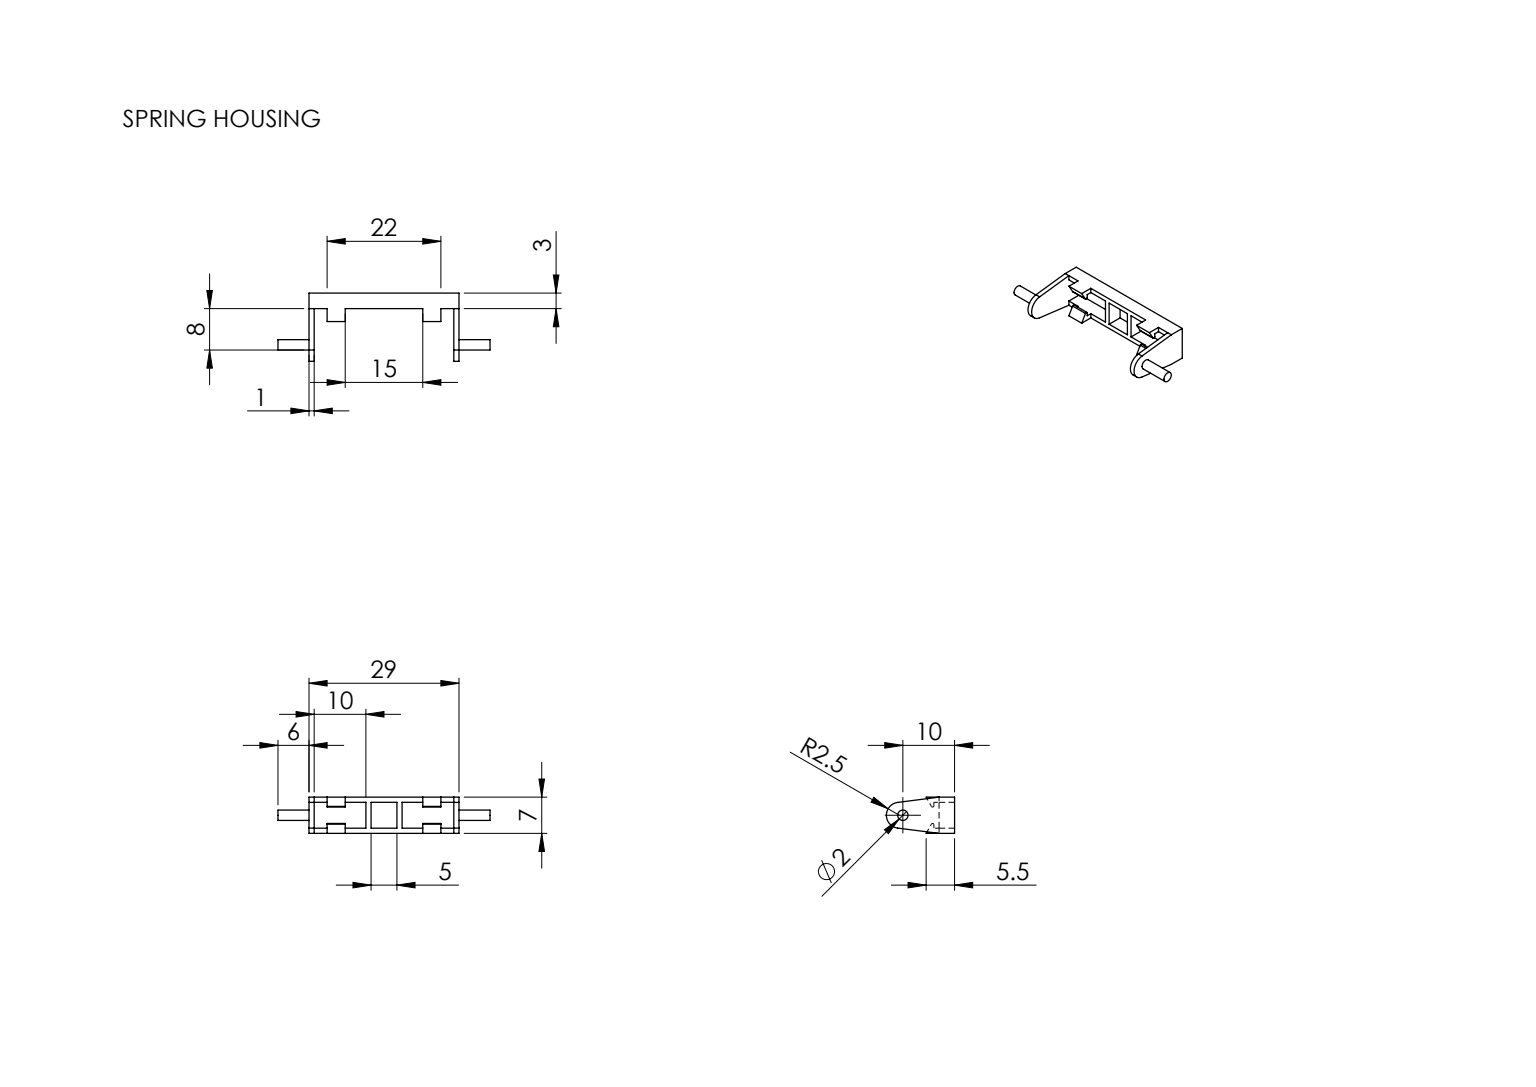
ISO-10303-21;
HEADER;
FILE_DESCRIPTION (('STEP AP214'),
    '1' );
FILE_NAME ('spring housing.step',
    '2026-10-04T16:38:04',
    ( '' ),
    ( '' ),
    'SwSTEP 2.0',
    'SolidWorks 2026',
    '' );
FILE_SCHEMA (( 'AUTOMOTIVE_DESIGN' ));
ENDSEC;

DATA;
#7=VECTOR ( 'NONE', #16168, 1000.000000000000000 ) ;
#16=CARTESIAN_POINT ( 'NONE',  ( -13.49999999999998401, -21.99999999999999645, 11.68378559369222280 ) ) ;
#34=ADVANCED_FACE ( 'NONE', ( #11140 ), #17508, .F. ) ;
#55=EDGE_CURVE ( 'NONE', #14709, #7180, #17615, .T. ) ;
#72=ORIENTED_EDGE ( 'NONE', *, *, #11352, .T. ) ;
#82=EDGE_CURVE ( 'NONE', #4544, #2802, #3495, .T. ) ;
#95=VERTEX_POINT ( 'NONE', #2332 ) ;
#103=LINE ( 'NONE', #17562, #12127 ) ;
#110=CARTESIAN_POINT ( 'NONE',  ( -11.00000000000000000, -25.49999999999999645, 6.500000000000000000 ) ) ;
#154=EDGE_CURVE ( 'NONE', #3175, #3359, #11545, .T. ) ;
#185=FILL_AREA_STYLE ('',( #1857 ) ) ;
#217=ORIENTED_EDGE ( 'NONE', *, *, #4935, .T. ) ;
#220=ORIENTED_EDGE ( 'NONE', *, *, #415, .T. ) ;
#228=DIRECTION ( 'NONE',  ( -0.000000000000000000, -0.000000000000000000, -1.000000000000000000 ) ) ;
#248=EDGE_LOOP ( 'NONE', ( #4182, #12799, #16047, #1135 ) ) ;
#267=ORIENTED_EDGE ( 'NONE', *, *, #11944, .F. ) ;
#268=ORIENTED_EDGE ( 'NONE', *, *, #5212, .F. ) ;
#281=EDGE_CURVE ( 'NONE', #9560, #10619, #19020, .T. ) ;
#292=ORIENTED_EDGE ( 'NONE', *, *, #13482, .F. ) ;
#293=EDGE_CURVE ( 'NONE', #3359, #13135, #6295, .T. ) ;
#296=ORIENTED_EDGE ( 'NONE', *, *, #17959, .F. ) ;
#315=AXIS2_PLACEMENT_3D ( 'NONE', #4243, #16683, #17105 ) ;
#321=CARTESIAN_POINT ( 'NONE',  ( -7.500000000000000000, -20.16506350946107418, 5.000000000000000000 ) ) ;
#332=CARTESIAN_POINT ( 'NONE',  ( -7.500000000000000000, -20.16506350946107418, 5.250000000000000000 ) ) ;
#339=EDGE_CURVE ( 'NONE', #9554, #1664, #7256, .T. ) ;
#354=CARTESIAN_POINT ( 'NONE',  ( -7.499999999999999112, -18.49999999999999645, 4.000000000000000000 ) ) ;
#362=VECTOR ( 'NONE', #20394, 1000.000000000000000 ) ;
#365=CARTESIAN_POINT ( 'NONE',  ( 7.499999999999999112, -23.83493649053891517, 5.249999999999999112 ) ) ;
#372=VECTOR ( 'NONE', #20232, 1000.000000000000000 ) ;
#380=CARTESIAN_POINT ( 'NONE',  ( -7.500000000000000000, -18.49999999999999645, 6.500000000000000888 ) ) ;
#390=DIRECTION ( 'NONE',  ( 0.000000000000000000, 1.000000000000000000, 0.000000000000000000 ) ) ;
#399=ORIENTED_EDGE ( 'NONE', *, *, #570, .F. ) ;
#403=ORIENTED_EDGE ( 'NONE', *, *, #20429, .T. ) ;
#415=EDGE_CURVE ( 'NONE', #11125, #7180, #2437, .T. ) ;
#422=AXIS2_PLACEMENT_3D ( 'NONE', #14755, #433, #5548 ) ;
#433=DIRECTION ( 'NONE',  ( 0.000000000000000000, -0.5000000000000041078, -0.8660254037844363761 ) ) ;
#438=DIRECTION ( 'NONE',  ( -1.000000000000000000, -0.000000000000000000, -0.000000000000000000 ) ) ;
#443=CARTESIAN_POINT ( 'NONE',  ( 11.00000000000000000, -25.49999999999999645, 6.500000000000000000 ) ) ;
#464=AXIS2_PLACEMENT_3D ( 'NONE', #5893, #7568, #2859 ) ;
#467=VECTOR ( 'NONE', #4908, 1000.000000000000000 ) ;
#482=ORIENTED_EDGE ( 'NONE', *, *, #7824, .T. ) ;
#483=VERTEX_POINT ( 'NONE', #11877 ) ;
#528=EDGE_CURVE ( 'NONE', #5816, #15348, #13237, .T. ) ;
#560=DIRECTION ( 'NONE',  ( -0.000000000000000000, 0.000000000000000000, -1.000000000000000000 ) ) ;
#566=EDGE_CURVE ( 'NONE', #17379, #995, #898, .T. ) ;
#570=EDGE_CURVE ( 'NONE', #2226, #5682, #13143, .T. ) ;
#596=CARTESIAN_POINT ( 'NONE',  ( 11.00000000000000000, -18.49999999999999645, 6.500000000000000888 ) ) ;
#608=EDGE_CURVE ( 'NONE', #4592, #5966, #18167, .T. ) ;
#623=DIRECTION ( 'NONE',  ( 0.000000000000000000, 1.000000000000000000, 0.000000000000000000 ) ) ;
#625=VECTOR ( 'NONE', #15350, 1000.000000000000000 ) ;
#635=CARTESIAN_POINT ( 'NONE',  ( -7.500000000000000000, -23.83493649053891517, 4.999999999999999112 ) ) ;
#637=ADVANCED_FACE ( 'NONE', ( #5502 ), #2365, .F. ) ;
#693=DIRECTION ( 'NONE',  ( 1.000000000000000000, 0.000000000000000000, 0.000000000000000000 ) ) ;
#694=CARTESIAN_POINT ( 'NONE',  ( -14.49999999999998579, -18.49999999999999645, 4.000000000000000000 ) ) ;
#716=VECTOR ( 'NONE', #3309, 1000.000000000000000 ) ;
#720=EDGE_CURVE ( 'NONE', #9416, #11125, #2883, .T. ) ;
#735=CARTESIAN_POINT ( 'NONE',  ( 7.499999999999999112, -18.49999999999999645, 6.500000000000000888 ) ) ;
#736=DIRECTION ( 'NONE',  ( 0.000000000000000000, 0.1264857625231113059, 0.9919684228235025047 ) ) ;
#739=CARTESIAN_POINT ( 'NONE',  ( -14.49999999999998579, -25.49999999999999645, 1.000000000000000000 ) ) ;
#741=EDGE_LOOP ( 'NONE', ( #10887, #4261, #18676, #2268, #15145, #1206, #20181, #1106, #10536, #17693, #14548, #16300, #9153, #18986 ) ) ;
#768=ORIENTED_EDGE ( 'NONE', *, *, #15761, .T. ) ;
#790=ORIENTED_EDGE ( 'NONE', *, *, #9633, .T. ) ;
#795=EDGE_CURVE ( 'NONE', #20584, #14806, #3312, .T. ) ;
#809=EDGE_CURVE ( 'NONE', #15986, #11334, #18580, .T. ) ;
#814=VERTEX_POINT ( 'NONE', #10623 ) ;
#838=CARTESIAN_POINT ( 'NONE',  ( -11.00000000000000000, -19.49999999999999645, 5.000000000000000000 ) ) ;
#840=ORIENTED_EDGE ( 'NONE', *, *, #2595, .T. ) ;
#842=VECTOR ( 'NONE', #18531, 1000.000000000000000 ) ;
#858=EDGE_CURVE ( 'NONE', #20067, #12385, #1217, .T. ) ;
#859=DIRECTION ( 'NONE',  ( -1.000000000000000000, 0.000000000000000000, 0.000000000000000000 ) ) ;
#863=ORIENTED_EDGE ( 'NONE', *, *, #1373, .F. ) ;
#867=EDGE_LOOP ( 'NONE', ( #4255, #16725 ) ) ;
#874=CARTESIAN_POINT ( 'NONE',  ( 11.00000000000000000, -24.49999999999999289, 5.000000000000000000 ) ) ;
#891=DIRECTION ( 'NONE',  ( -1.000000000000000000, 0.000000000000000000, 0.000000000000000000 ) ) ;
#896=DIRECTION ( 'NONE',  ( -1.000000000000000000, -0.000000000000000000, -0.000000000000000000 ) ) ;
#898=LINE ( 'NONE', #2062, #2292 ) ;
#914=ORIENTED_EDGE ( 'NONE', *, *, #3010, .F. ) ;
#923=CYLINDRICAL_SURFACE ( 'NONE', #19544, 2.500000000000000444 ) ;
#926=ADVANCED_FACE ( 'NONE', ( #14369 ), #17418, .T. ) ;
#938=LINE ( 'NONE', #739, #9319 ) ;
#948=CARTESIAN_POINT ( 'NONE',  ( 11.00000000000000000, -20.29006350946107418, 5.466506350946110260 ) ) ;
#950=LINE ( 'NONE', #5663, #9851 ) ;
#957=CARTESIAN_POINT ( 'NONE',  ( -11.00000000000000000, -19.49999999999999645, 5.000000000000000000 ) ) ;
#968=VECTOR ( 'NONE', #2534, 1000.000000000000000 ) ;
#973=VECTOR ( 'NONE', #693, 1000.000000000000000 ) ;
#979=CARTESIAN_POINT ( 'NONE',  ( 11.00000000000000000, -18.49999999999999645, 4.000000000000000000 ) ) ;
#987=ADVANCED_FACE ( 'NONE', ( #3397 ), #11143, .F. ) ;
#993=DIRECTION ( 'NONE',  ( -1.000000000000000000, -0.000000000000000000, -0.000000000000000000 ) ) ;
#995=VERTEX_POINT ( 'NONE', #20668 ) ;
#1009=CARTESIAN_POINT ( 'NONE',  ( 7.499999999999999112, -24.49999999999999289, 4.000000000000000000 ) ) ;
#1025=ORIENTED_EDGE ( 'NONE', *, *, #18401, .F. ) ;
#1030=EDGE_CURVE ( 'NONE', #9195, #15413, #4961, .T. ) ;
#1056=( NAMED_UNIT ( * ) PLANE_ANGLE_UNIT ( ) SI_UNIT ( $, .RADIAN. ) );
#1067=LINE ( 'NONE', #9213, #14396 ) ;
#1096=ORIENTED_EDGE ( 'NONE', *, *, #15655, .F. ) ;
#1098=CARTESIAN_POINT ( 'NONE',  ( -13.49999999999998401, -24.49999999999999289, 4.000000000000000000 ) ) ;
#1106=ORIENTED_EDGE ( 'NONE', *, *, #14014, .T. ) ;
#1107=ORIENTED_EDGE ( 'NONE', *, *, #8472, .T. ) ;
#1118=DIRECTION ( 'NONE',  ( -1.000000000000000000, 0.000000000000000000, 0.000000000000000000 ) ) ;
#1120=CARTESIAN_POINT ( 'NONE',  ( -14.49999999999998579, -18.49999999999999645, 4.000000000000000000 ) ) ;
#1122=AXIS2_PLACEMENT_3D ( 'NONE', #3753, #9921, #5424 ) ;
#1135=ORIENTED_EDGE ( 'NONE', *, *, #13755, .F. ) ;
#1158=CARTESIAN_POINT ( 'NONE',  ( -3.499999999999997780, -24.49999999999999289, 4.000000000000000000 ) ) ;
#1159=ORIENTED_EDGE ( 'NONE', *, *, #7829, .F. ) ;
#1160=DIRECTION ( 'NONE',  ( 1.000000000000000000, -0.000000000000000000, -0.000000000000000000 ) ) ;
#1162=CARTESIAN_POINT ( 'NONE',  ( 13.49999999999998401, -21.99999999999999645, 11.68378559369222280 ) ) ;
#1177=ORIENTED_EDGE ( 'NONE', *, *, #15399, .T. ) ;
#1180=VERTEX_POINT ( 'NONE', #19610 ) ;
#1191=CARTESIAN_POINT ( 'NONE',  ( -14.49999999999998579, -25.49999999999999645, 4.000000000000000000 ) ) ;
#1192=LINE ( 'NONE', #9038, #12638 ) ;
#1203=ORIENTED_EDGE ( 'NONE', *, *, #15128, .F. ) ;
#1205=DIRECTION ( 'NONE',  ( -0.000000000000000000, 0.1264857625231113059, -0.9919684228235025047 ) ) ;
#1206=ORIENTED_EDGE ( 'NONE', *, *, #9633, .F. ) ;
#1212=CARTESIAN_POINT ( 'NONE',  ( 13.49999999999998401, -19.52007894294123957, 12.00000000000000000 ) ) ;
#1214=CARTESIAN_POINT ( 'NONE',  ( -14.49999999999998579, -18.49999999999999645, 1.000000000000000000 ) ) ;
#1217=LINE ( 'NONE', #13958, #17678 ) ;
#1232=LINE ( 'NONE', #7714, #19995 ) ;
#1233=ORIENTED_EDGE ( 'NONE', *, *, #720, .F. ) ;
#1243=CARTESIAN_POINT ( 'NONE',  ( 13.49999999999998401, -24.47992105705875332, 12.00000000000000000 ) ) ;
#1263=ORIENTED_EDGE ( 'NONE', *, *, #16479, .T. ) ;
#1292=LINE ( 'NONE', #7570, #4387 ) ;
#1303=VECTOR ( 'NONE', #14815, 1000.000000000000000 ) ;
#1307=CYLINDRICAL_SURFACE ( 'NONE', #12478, 1.000000000000002665 ) ;
#1308=EDGE_CURVE ( 'NONE', #16594, #7416, #10706, .T. ) ;
#1310=VERTEX_POINT ( 'NONE', #2758 ) ;
#1324=VECTOR ( 'NONE', #8795, 1000.000000000000000 ) ;
#1326=CARTESIAN_POINT ( 'NONE',  ( -7.499999999999999112, -18.49999999999999645, 6.500000000000000888 ) ) ;
#1327=DIRECTION ( 'NONE',  ( -1.000000000000000000, 0.000000000000000000, 0.000000000000000000 ) ) ;
#1360=EDGE_CURVE ( 'NONE', #5898, #18235, #5688, .T. ) ;
#1362=EDGE_CURVE ( 'NONE', #8225, #1180, #13727, .T. ) ;
#1373=EDGE_CURVE ( 'NONE', #17295, #15081, #2438, .T. ) ;
#1376=DIRECTION ( 'NONE',  ( -1.000000000000000000, -0.000000000000000000, -0.000000000000000000 ) ) ;
#1390=DIRECTION ( 'NONE',  ( 1.000000000000000000, 0.000000000000000000, -0.000000000000000000 ) ) ;
#1395=CARTESIAN_POINT ( 'NONE',  ( -14.49999999999998579, -21.99999999999999645, 11.68378559369222280 ) ) ;
#1403=EDGE_LOOP ( 'NONE', ( #8385, #4546, #1263, #5932 ) ) ;
#1413=ORIENTED_EDGE ( 'NONE', *, *, #8902, .T. ) ;
#1443=VERTEX_POINT ( 'NONE', #874 ) ;
#1461=VERTEX_POINT ( 'NONE', #20548 ) ;
#1463=ORIENTED_EDGE ( 'NONE', *, *, #2388, .F. ) ;
#1485=ORIENTED_EDGE ( 'NONE', *, *, #20231, .F. ) ;
#1487=ORIENTED_EDGE ( 'NONE', *, *, #4376, .F. ) ;
#1492=EDGE_CURVE ( 'NONE', #8225, #19576, #11119, .T. ) ;
#1495=CARTESIAN_POINT ( 'NONE',  ( -20.49999999999998224, -21.99999999999999645, 11.00000000000000178 ) ) ;
#1505=ORIENTED_EDGE ( 'NONE', *, *, #18166, .T. ) ;
#1508=CARTESIAN_POINT ( 'NONE',  ( 11.00000000000000000, -23.83493649053891517, 4.999999999999999112 ) ) ;
#1514=DIRECTION ( 'NONE',  ( 1.000000000000000000, 0.000000000000000000, 0.000000000000000000 ) ) ;
#1534=ORIENTED_EDGE ( 'NONE', *, *, #3010, .T. ) ;
#1538=EDGE_CURVE ( 'NONE', #2967, #1461, #17489, .T. ) ;
#1553=ORIENTED_EDGE ( 'NONE', *, *, #6829, .T. ) ;
#1554=AXIS2_PLACEMENT_3D ( 'NONE', #19099, #8305, #11236 ) ;
#1570=EDGE_CURVE ( 'NONE', #1664, #16077, #9543, .T. ) ;
#1575=CARTESIAN_POINT ( 'NONE',  ( -14.49999999999998579, -25.49999999999999645, 4.000000000000000000 ) ) ;
#1582=PLANE ( 'NONE',  #7681 ) ;
#1596=EDGE_CURVE ( 'NONE', #2802, #18601, #3387, .T. ) ;
#1616=DIRECTION ( 'NONE',  ( 0.000000000000000000, 0.000000000000000000, 1.000000000000000000 ) ) ;
#1627=VECTOR ( 'NONE', #3594, 1000.000000000000000 ) ;
#1639=CARTESIAN_POINT ( 'NONE',  ( 7.499999999999999112, -20.16506350946107418, 5.000000000000000000 ) ) ;
#1650=DIRECTION ( 'NONE',  ( 0.000000000000000000, 0.1264857625231113059, 0.9919684228235025047 ) ) ;
#1654=CARTESIAN_POINT ( 'NONE',  ( 11.00000000000000000, -18.49999999999999645, 6.500000000000000888 ) ) ;
#1663=VECTOR ( 'NONE', #13515, 1000.000000000000000 ) ;
#1664=VERTEX_POINT ( 'NONE', #443 ) ;
#1669=CARTESIAN_POINT ( 'NONE',  ( 11.00000000000000000, -20.16506350946107418, 5.000000000000000000 ) ) ;
#1698=DIRECTION ( 'NONE',  ( -1.000000000000000000, 0.000000000000000000, 0.000000000000000000 ) ) ;
#1709=EDGE_CURVE ( 'NONE', #17379, #20661, #13091, .T. ) ;
#1713=CARTESIAN_POINT ( 'NONE',  ( 13.49999999999998401, -19.52007894294123957, 12.00000000000000000 ) ) ;
#1724=CARTESIAN_POINT ( 'NONE',  ( 7.499999999999999112, -23.83493649053891517, 4.999999999999999112 ) ) ;
#1732=EDGE_CURVE ( 'NONE', #3797, #7379, #13191, .T. ) ;
#1771=CIRCLE ( 'NONE', #7777, 1.000000000000002665 ) ;
#1785=DIRECTION ( 'NONE',  ( 0.000000000000000000, 0.000000000000000000, 1.000000000000000000 ) ) ;
#1790=ORIENTED_EDGE ( 'NONE', *, *, #11684, .T. ) ;
#1793=CARTESIAN_POINT ( 'NONE',  ( 0.000000000000000000, 0.000000000000000000, 0.000000000000000000 ) ) ;
#1797=CARTESIAN_POINT ( 'NONE',  ( 14.50000000000001243, -18.49999999999999645, 1.000000000000000000 ) ) ;
#1803=DIRECTION ( 'NONE',  ( -1.000000000000000000, -0.000000000000000000, -0.000000000000000000 ) ) ;
#1806=EDGE_CURVE ( 'NONE', #3359, #14333, #8700, .T. ) ;
#1823=DIRECTION ( 'NONE',  ( -0.000000000000000000, 0.000000000000000000, 1.000000000000000000 ) ) ;
#1824=ORIENTED_EDGE ( 'NONE', *, *, #16454, .T. ) ;
#1826=CARTESIAN_POINT ( 'NONE',  ( 11.00000000000000000, -20.16506350946107418, 5.000000000000000000 ) ) ;
#1836=ORIENTED_EDGE ( 'NONE', *, *, #5658, .T. ) ;
#1857=FILL_AREA_STYLE_COLOUR ( '', #17300 ) ;
#1859=PLANE ( 'NONE',  #6196 ) ;
#1871=ORIENTED_EDGE ( 'NONE', *, *, #10640, .F. ) ;
#1888=PLANE ( 'NONE',  #11720 ) ;
#1899=CARTESIAN_POINT ( 'NONE',  ( -13.49999999999998401, -21.99999999999999645, 14.18378559369222280 ) ) ;
#1910=AXIS2_PLACEMENT_3D ( 'NONE', #9537, #3065, #12980 ) ;
#1912=DIRECTION ( 'NONE',  ( 1.734723475976809560E-16, -1.000000000000000000, 0.000000000000000000 ) ) ;
#1923=PLANE ( 'NONE',  #2904 ) ;
#1929=AXIS2_PLACEMENT_3D ( 'NONE', #10642, #15450, #16810 ) ;
#1941=DIRECTION ( 'NONE',  ( -0.000000000000000000, -0.8660254037844364872, -0.5000000000000036637 ) ) ;
#1950=VECTOR ( 'NONE', #12612, 1000.000000000000000 ) ;
#1958=SURFACE_SIDE_STYLE ('',( #8035 ) ) ;
#1960=DIRECTION ( 'NONE',  ( -0.000000000000000000, 0.000000000000000000, -1.000000000000000000 ) ) ;
#1974=AXIS2_PLACEMENT_3D ( 'NONE', #12021, #11711, #18107 ) ;
#1977=EDGE_CURVE ( 'NONE', #7180, #17356, #1067, .T. ) ;
#1996=ORIENTED_EDGE ( 'NONE', *, *, #15355, .T. ) ;
#1998=DIRECTION ( 'NONE',  ( -0.000000000000000000, -0.000000000000000000, -1.000000000000000000 ) ) ;
#2013=FACE_BOUND ( 'NONE', #12922, .T. ) ;
#2029=LINE ( 'NONE', #8418, #8249 ) ;
#2037=VECTOR ( 'NONE', #17601, 1000.000000000000000 ) ;
#2049=ORIENTED_EDGE ( 'NONE', *, *, #17282, .T. ) ;
#2054=DIRECTION ( 'NONE',  ( -1.000000000000000000, -0.000000000000000000, -0.000000000000000000 ) ) ;
#2062=CARTESIAN_POINT ( 'NONE',  ( 7.500000000000000000, -19.49999999999999645, 4.000000000000000000 ) ) ;
#2082=ORIENTED_EDGE ( 'NONE', *, *, #12798, .F. ) ;
#2087=CARTESIAN_POINT ( 'NONE',  ( 0.000000000000000000, 0.000000000000000000, 1.000000000000000000 ) ) ;
#2089=DIRECTION ( 'NONE',  ( -1.000000000000000000, -0.000000000000000000, -0.000000000000000000 ) ) ;
#2102=CARTESIAN_POINT ( 'NONE',  ( -11.00000000000000000, -23.83493649053891517, 4.999999999999999112 ) ) ;
#2109=EDGE_CURVE ( 'NONE', #13777, #3840, #4508, .T. ) ;
#2116=CARTESIAN_POINT ( 'NONE',  ( -14.49999999999998579, -21.99999999999999645, 11.68378559369222280 ) ) ;
#2127=VERTEX_POINT ( 'NONE', #9728 ) ;
#2130=PLANE ( 'NONE',  #19291 ) ;
#2136=CARTESIAN_POINT ( 'NONE',  ( 7.499999999999999112, -19.49999999999999645, 4.000000000000000000 ) ) ;
#2157=CYLINDRICAL_SURFACE ( 'NONE', #20022, 2.500000000000000444 ) ;
#2171=EDGE_CURVE ( 'NONE', #5966, #15986, #11290, .T. ) ;
#2176=DIRECTION ( 'NONE',  ( -0.000000000000000000, -1.000000000000000000, 0.000000000000000000 ) ) ;
#2178=CIRCLE ( 'NONE', #12865, 1.000000000000002665 ) ;
#2186=CARTESIAN_POINT ( 'NONE',  ( -14.49999999999998579, -21.99999999999999645, 11.00000000000000178 ) ) ;
#2190=LINE ( 'NONE', #10147, #4721 ) ;
#2203=EDGE_CURVE ( 'NONE', #17464, #10229, #7754, .T. ) ;
#2208=CARTESIAN_POINT ( 'NONE',  ( 11.00000000000000000, -20.16506350946107418, 5.250000000000000000 ) ) ;
#2226=VERTEX_POINT ( 'NONE', #110 ) ;
#2232=DIRECTION ( 'NONE',  ( 0.000000000000000000, -0.1264857625231113059, 0.9919684228235025047 ) ) ;
#2250=ORIENTED_EDGE ( 'NONE', *, *, #19877, .T. ) ;
#2255=CARTESIAN_POINT ( 'NONE',  ( -11.00000000000000000, -20.16506350946107418, 5.000000000000000000 ) ) ;
#2268=ORIENTED_EDGE ( 'NONE', *, *, #2171, .F. ) ;
#2270=PLANE ( 'NONE',  #1929 ) ;
#2275=ORIENTED_EDGE ( 'NONE', *, *, #1977, .F. ) ;
#2292=VECTOR ( 'NONE', #11978, 1000.000000000000000 ) ;
#2296=VERTEX_POINT ( 'NONE', #5326 ) ;
#2297=VERTEX_POINT ( 'NONE', #3653 ) ;
#2301=CARTESIAN_POINT ( 'NONE',  ( -14.49999999999998579, -24.49999999999999289, 4.000000000000000000 ) ) ;
#2330=VECTOR ( 'NONE', #7851, 1000.000000000000000 ) ;
#2332=CARTESIAN_POINT ( 'NONE',  ( -7.499999999999999112, -24.49999999999999289, 4.000000000000000000 ) ) ;
#2352=EDGE_CURVE ( 'NONE', #14282, #12772, #12019, .T. ) ;
#2362=EDGE_CURVE ( 'NONE', #12874, #9416, #3451, .T. ) ;
#2365=PLANE ( 'NONE',  #17326 ) ;
#2367=DIRECTION ( 'NONE',  ( 1.000000000000000000, 0.000000000000000000, 0.000000000000000000 ) ) ;
#2385=ORIENTED_EDGE ( 'NONE', *, *, #2109, .F. ) ;
#2388=EDGE_CURVE ( 'NONE', #814, #18396, #10689, .T. ) ;
#2393=CARTESIAN_POINT ( 'NONE',  ( -13.49999999999998401, -19.52007894294123957, 12.00000000000000000 ) ) ;
#2394=CARTESIAN_POINT ( 'NONE',  ( 13.50000000000001243, -18.49999999999999645, 4.000000000000000000 ) ) ;
#2400=DIRECTION ( 'NONE',  ( 0.000000000000000000, -0.8660254037844363761, 0.5000000000000041078 ) ) ;
#2430=CARTESIAN_POINT ( 'NONE',  ( 20.49999999999998224, -21.99999999999999645, 9.999999999999998224 ) ) ;
#2434=DIRECTION ( 'NONE',  ( 1.000000000000000000, 0.000000000000000000, -0.000000000000000000 ) ) ;
#2437=LINE ( 'NONE', #15195, #968 ) ;
#2438=LINE ( 'NONE', #18867, #372 ) ;
#2456=ADVANCED_FACE ( 'NONE', ( #19567 ), #8167, .T. ) ;
#2457=ORIENTED_EDGE ( 'NONE', *, *, #4151, .T. ) ;
#2484=DIRECTION ( 'NONE',  ( 0.000000000000000000, 1.000000000000000000, 0.000000000000000000 ) ) ;
#2494=PLANE ( 'NONE',  #20651 ) ;
#2495=CARTESIAN_POINT ( 'NONE',  ( 11.00000000000000000, -24.49999999999999289, 5.000000000000000000 ) ) ;
#2510=CARTESIAN_POINT ( 'NONE',  ( -14.49999999999998579, -24.49999999999999289, 1.000000000000000000 ) ) ;
#2512=VECTOR ( 'NONE', #15224, 1000.000000000000000 ) ;
#2515=ADVANCED_FACE ( 'NONE', ( #16604 ), #7212, .T. ) ;
#2534=DIRECTION ( 'NONE',  ( -0.000000000000000000, -0.000000000000000000, -1.000000000000000000 ) ) ;
#2561=ORIENTED_EDGE ( 'NONE', *, *, #16454, .F. ) ;
#2569=CARTESIAN_POINT ( 'NONE',  ( -14.49999999999998579, -19.49999999999999645, 4.000000000000000000 ) ) ;
#2585=ORIENTED_EDGE ( 'NONE', *, *, #14183, .T. ) ;
#2587=ORIENTED_EDGE ( 'NONE', *, *, #10224, .T. ) ;
#2595=EDGE_CURVE ( 'NONE', #7178, #9560, #20082, .T. ) ;
#2602=DIRECTION ( 'NONE',  ( 0.000000000000000000, 0.8660254037844363761, -0.5000000000000041078 ) ) ;
#2612=VECTOR ( 'NONE', #15562, 1000.000000000000000 ) ;
#2613=DIRECTION ( 'NONE',  ( 0.000000000000000000, 0.000000000000000000, -1.000000000000000000 ) ) ;
#2623=AXIS2_PLACEMENT_3D ( 'NONE', #3905, #10283, #16654 ) ;
#2627=CIRCLE ( 'NONE', #16989, 0.2500000000000002220 ) ;
#2641=VECTOR ( 'NONE', #4244, 1000.000000000000114 ) ;
#2648=CARTESIAN_POINT ( 'NONE',  ( 2.499999999999998668, -19.49999999999999645, 4.000000000000000000 ) ) ;
#2673=DIRECTION ( 'NONE',  ( 0.000000000000000000, 0.000000000000000000, -1.000000000000000000 ) ) ;
#2680=VECTOR ( 'NONE', #5272, 1000.000000000000000 ) ;
#2694=CARTESIAN_POINT ( 'NONE',  ( 2.499999999999998668, -19.50000000000000000, 1.000000000000000000 ) ) ;
#2703=EDGE_CURVE ( 'NONE', #14026, #15081, #10766, .T. ) ;
#2715=DIRECTION ( 'NONE',  ( 1.000000000000000000, 0.000000000000000000, -0.000000000000000000 ) ) ;
#2742=VECTOR ( 'NONE', #6065, 1000.000000000000227 ) ;
#2758=CARTESIAN_POINT ( 'NONE',  ( 13.50000000000001243, -24.49999999999999289, 1.000000000000000000 ) ) ;
#2765=ORIENTED_EDGE ( 'NONE', *, *, #9898, .T. ) ;
#2778=ORIENTED_EDGE ( 'NONE', *, *, #293, .F. ) ;
#2785=FACE_BOUND ( 'NONE', #9102, .T. ) ;
#2802=VERTEX_POINT ( 'NONE', #13122 ) ;
#2815=DIRECTION ( 'NONE',  ( 0.000000000000000000, 0.8660254037844364872, 0.5000000000000036637 ) ) ;
#2825=EDGE_LOOP ( 'NONE', ( #1203, #14184, #13332, #8079, #16097, #14135 ) ) ;
#2826=ORIENTED_EDGE ( 'NONE', *, *, #17610, .T. ) ;
#2859=DIRECTION ( 'NONE',  ( 0.000000000000000000, 0.000000000000000000, -1.000000000000000000 ) ) ;
#2861=EDGE_CURVE ( 'NONE', #14282, #483, #9781, .T. ) ;
#2865=EDGE_LOOP ( 'NONE', ( #2826, #2049, #1487, #13747 ) ) ;
#2870=ORIENTED_EDGE ( 'NONE', *, *, #2861, .F. ) ;
#2883=LINE ( 'NONE', #12188, #6992 ) ;
#2896=EDGE_CURVE ( 'NONE', #20148, #17464, #8426, .T. ) ;
#2904=AXIS2_PLACEMENT_3D ( 'NONE', #3090, #1823, #1514 ) ;
#2919=LINE ( 'NONE', #4586, #17101 ) ;
#2946=FACE_OUTER_BOUND ( 'NONE', #3035, .T. ) ;
#2949=ORIENTED_EDGE ( 'NONE', *, *, #3053, .F. ) ;
#2960=CYLINDRICAL_SURFACE ( 'NONE', #3344, 1.000000000000002665 ) ;
#2967=VERTEX_POINT ( 'NONE', #1797 ) ;
#2985=ORIENTED_EDGE ( 'NONE', *, *, #1362, .F. ) ;
#2988=AXIS2_PLACEMENT_3D ( 'NONE', #3732, #13144, #11263 ) ;
#2992=CARTESIAN_POINT ( 'NONE',  ( 11.00000000000000000, -19.49999999999999645, 4.000000000000000000 ) ) ;
#2995=DIRECTION ( 'NONE',  ( -1.000000000000000000, -0.000000000000000000, -0.000000000000000000 ) ) ;
#3010=EDGE_CURVE ( 'NONE', #11512, #8225, #8280, .T. ) ;
#3016=AXIS2_PLACEMENT_3D ( 'NONE', #2394, #10656, #18716 ) ;
#3021=VECTOR ( 'NONE', #1650, 1000.000000000000227 ) ;
#3027=DIRECTION ( 'NONE',  ( -0.000000000000000000, 0.000000000000000000, -1.000000000000000000 ) ) ;
#3034=CARTESIAN_POINT ( 'NONE',  ( 11.00000000000000000, -23.83493649053891517, 5.249999999999999112 ) ) ;
#3035=EDGE_LOOP ( 'NONE', ( #2082, #7589, #3333, #14527 ) ) ;
#3038=EDGE_CURVE ( 'NONE', #2127, #18601, #16130, .T. ) ;
#3053=EDGE_CURVE ( 'NONE', #5903, #4592, #11310, .T. ) ;
#3055=LINE ( 'NONE', #15801, #10085 ) ;
#3061=VERTEX_POINT ( 'NONE', #14652 ) ;
#3065=DIRECTION ( 'NONE',  ( -1.000000000000000000, -0.000000000000000000, -0.000000000000000000 ) ) ;
#3068=DIRECTION ( 'NONE',  ( -0.000000000000000000, -0.000000000000000000, -1.000000000000000000 ) ) ;
#3078=DIRECTION ( 'NONE',  ( 0.000000000000000000, -0.1264857625231113059, -0.9919684228235025047 ) ) ;
#3090=CARTESIAN_POINT ( 'NONE',  ( 0.000000000000000000, 0.000000000000000000, 4.000000000000000000 ) ) ;
#3105=EDGE_CURVE ( 'NONE', #13135, #11513, #19380, .T. ) ;
#3109=LINE ( 'NONE', #7816, #19369 ) ;
#3121=CARTESIAN_POINT ( 'NONE',  ( -13.49999999999998401, -25.49999999999999645, 4.000000000000000000 ) ) ;
#3123=CARTESIAN_POINT ( 'NONE',  ( -14.49999999999998579, -19.49999999999999645, 4.000000000000000000 ) ) ;
#3139=AXIS2_PLACEMENT_3D ( 'NONE', #10187, #16557, #2232 ) ;
#3162=ORIENTED_EDGE ( 'NONE', *, *, #9798, .F. ) ;
#3163=CARTESIAN_POINT ( 'NONE',  ( -7.500000000000000000, -20.29006350946107418, 5.466506350946110260 ) ) ;
#3175=VERTEX_POINT ( 'NONE', #14760 ) ;
#3180=ORIENTED_EDGE ( 'NONE', *, *, #17282, .F. ) ;
#3187=AXIS2_PLACEMENT_3D ( 'NONE', #9363, #16628, #4194 ) ;
#3195=DIRECTION ( 'NONE',  ( 1.000000000000000000, 8.673617379884045333E-17, -0.000000000000000000 ) ) ;
#3206=ORIENTED_EDGE ( 'NONE', *, *, #7111, .F. ) ;
#3231=DIRECTION ( 'NONE',  ( 0.000000000000000000, -1.000000000000000000, 0.000000000000000000 ) ) ;
#3261=CYLINDRICAL_SURFACE ( 'NONE', #1910, 1.000000000000002665 ) ;
#3272=ORIENTED_EDGE ( 'NONE', *, *, #339, .F. ) ;
#3285=AXIS2_PLACEMENT_3D ( 'NONE', #18381, #18068, #2367 ) ;
#3286=CARTESIAN_POINT ( 'NONE',  ( 11.00000000000000000, -23.83493649053891517, 5.249999999999999112 ) ) ;
#3295=AXIS2_PLACEMENT_3D ( 'NONE', #17829, #13417, #14883 ) ;
#3296=CIRCLE ( 'NONE', #5975, 1.000000000000002665 ) ;
#3309=DIRECTION ( 'NONE',  ( -0.000000000000000000, -1.000000000000000000, 0.000000000000000000 ) ) ;
#3312=CIRCLE ( 'NONE', #4652, 1.000000000000002665 ) ;
#3315=DIRECTION ( 'NONE',  ( -1.000000000000000000, 0.000000000000000000, 0.000000000000000000 ) ) ;
#3324=ORIENTED_EDGE ( 'NONE', *, *, #20088, .T. ) ;
#3332=CIRCLE ( 'NONE', #11346, 2.500000000000000444 ) ;
#3333=ORIENTED_EDGE ( 'NONE', *, *, #2896, .T. ) ;
#3336=ORIENTED_EDGE ( 'NONE', *, *, #17550, .T. ) ;
#3344=AXIS2_PLACEMENT_3D ( 'NONE', #1495, #20449, #14143 ) ;
#3359=VERTEX_POINT ( 'NONE', #635 ) ;
#3387=CIRCLE ( 'NONE', #19421, 2.500000000000000444 ) ;
#3395=VERTEX_POINT ( 'NONE', #15064 ) ;
#3397=FACE_OUTER_BOUND ( 'NONE', #13302, .T. ) ;
#3414=ORIENTED_EDGE ( 'NONE', *, *, #10183, .T. ) ;
#3416=CARTESIAN_POINT ( 'NONE',  ( -3.499999999999997780, -19.49999999999999645, 4.000000000000000000 ) ) ;
#3420=ORIENTED_EDGE ( 'NONE', *, *, #720, .T. ) ;
#3437=VERTEX_POINT ( 'NONE', #1326 ) ;
#3439=CARTESIAN_POINT ( 'NONE',  ( 2.499999999999999112, -24.49999999999999289, 1.000000000000000000 ) ) ;
#3448=PLANE ( 'NONE',  #14464 ) ;
#3451=LINE ( 'NONE', #3861, #20059 ) ;
#3456=LINE ( 'NONE', #14636, #18079 ) ;
#3461=ORIENTED_EDGE ( 'NONE', *, *, #13218, .T. ) ;
#3482=EDGE_CURVE ( 'NONE', #1664, #11612, #15539, .T. ) ;
#3494=CARTESIAN_POINT ( 'NONE',  ( 14.50000000000001243, -25.49999999999999645, 4.000000000000000000 ) ) ;
#3495=LINE ( 'NONE', #9974, #10646 ) ;
#3501=CARTESIAN_POINT ( 'NONE',  ( -14.49999999999998579, -19.49999999999999645, 1.000000000000000000 ) ) ;
#3511=AXIS2_PLACEMENT_3D ( 'NONE', #2208, #15069, #8590 ) ;
#3530=LINE ( 'NONE', #3123, #3940 ) ;
#3532=CARTESIAN_POINT ( 'NONE',  ( 11.00000000000000000, -20.16506350946107418, 5.250000000000000000 ) ) ;
#3538=ORIENTED_EDGE ( 'NONE', *, *, #2203, .T. ) ;
#3541=ORIENTED_EDGE ( 'NONE', *, *, #10425, .T. ) ;
#3544=PLANE ( 'NONE',  #1122 ) ;
#3556=PLANE ( 'NONE',  #8080 ) ;
#3594=DIRECTION ( 'NONE',  ( 0.000000000000000000, 1.000000000000000000, -1.304178812473495102E-15 ) ) ;
#3610=CARTESIAN_POINT ( 'NONE',  ( -11.00000000000000000, -23.70993649053891517, 5.466506350946108483 ) ) ;
#3613=CARTESIAN_POINT ( 'NONE',  ( 7.499999999999999112, -18.49999999999999645, 4.000000000000000000 ) ) ;
#3643=SHAPE_DEFINITION_REPRESENTATION ( #5005, #6161 ) ;
#3653=CARTESIAN_POINT ( 'NONE',  ( -2.499999999999998668, -24.49999999999999289, 4.000000000000000000 ) ) ;
#3668=DIRECTION ( 'NONE',  ( 1.734723475976809560E-16, -1.000000000000000000, 0.000000000000000000 ) ) ;
#3672=VECTOR ( 'NONE', #7591, 1000.000000000000000 ) ;
#3697=ORIENTED_EDGE ( 'NONE', *, *, #7459, .F. ) ;
#3698=EDGE_LOOP ( 'NONE', ( #10786, #8846, #17765, #2870 ) ) ;
#3732=CARTESIAN_POINT ( 'NONE',  ( 11.00000000000000000, -23.83493649053891517, 4.999999999999999112 ) ) ;
#3751=VERTEX_POINT ( 'NONE', #6113 ) ;
#3753=CARTESIAN_POINT ( 'NONE',  ( -11.00000000000000000, -23.83493649053891517, 5.249999999999999112 ) ) ;
#3759=CARTESIAN_POINT ( 'NONE',  ( -14.49999999999998579, -19.49999999999999645, 1.000000000000000000 ) ) ;
#3769=AXIS2_PLACEMENT_3D ( 'NONE', #9130, #2434, #5887 ) ;
#3775=DIRECTION ( 'NONE',  ( 0.000000000000000000, 0.000000000000000000, -1.000000000000000000 ) ) ;
#3797=VERTEX_POINT ( 'NONE', #1098 ) ;
#3800=DIRECTION ( 'NONE',  ( -0.000000000000000000, -0.8660254037844363761, 0.5000000000000041078 ) ) ;
#3809=PLANE ( 'NONE',  #3139 ) ;
#3815=ORIENTED_EDGE ( 'NONE', *, *, #12646, .T. ) ;
#3825=FACE_OUTER_BOUND ( 'NONE', #867, .T. ) ;
#3831=FACE_OUTER_BOUND ( 'NONE', #4590, .T. ) ;
#3840=VERTEX_POINT ( 'NONE', #20142 ) ;
#3857=DIRECTION ( 'NONE',  ( -0.000000000000000000, -0.000000000000000000, 1.000000000000000000 ) ) ;
#3861=CARTESIAN_POINT ( 'NONE',  ( -14.49999999999998579, -18.49999999999999645, 4.000000000000000000 ) ) ;
#3873=PLANE ( 'NONE',  #422 ) ;
#3886=FACE_OUTER_BOUND ( 'NONE', #6170, .T. ) ;
#3900=ADVANCED_FACE ( 'NONE', ( #5900 ), #12270, .T. ) ;
#3905=CARTESIAN_POINT ( 'NONE',  ( -7.500000000000000000, -23.83493649053891517, 5.249999999999999112 ) ) ;
#3914=ORIENTED_EDGE ( 'NONE', *, *, #2703, .T. ) ;
#3932=FACE_OUTER_BOUND ( 'NONE', #14417, .T. ) ;
#3933=ADVANCED_FACE ( 'NONE', ( #9145 ), #6005, .T. ) ;
#3940=VECTOR ( 'NONE', #9905, 1000.000000000000000 ) ;
#3947=CARTESIAN_POINT ( 'NONE',  ( 11.00000000000000000, -20.16506350946107418, 5.000000000000000000 ) ) ;
#3953=DIRECTION ( 'NONE',  ( 0.000000000000000000, 0.000000000000000000, 1.000000000000000000 ) ) ;
#3964=DIRECTION ( 'NONE',  ( -0.000000000000000000, 0.000000000000000000, -1.000000000000000000 ) ) ;
#3965=DIRECTION ( 'NONE',  ( 0.000000000000000000, -0.5000000000000041078, -0.8660254037844363761 ) ) ;
#3970=LINE ( 'NONE', #838, #1324 ) ;
#3976=VECTOR ( 'NONE', #2484, 1000.000000000000000 ) ;
#3978=FILL_AREA_STYLE_COLOUR ( '', #19719 ) ;
#3994=CARTESIAN_POINT ( 'NONE',  ( -14.49999999999998579, -19.49999999999999645, 4.000000000000000000 ) ) ;
#4007=DIRECTION ( 'NONE',  ( -1.000000000000000000, 0.000000000000000000, 0.000000000000000000 ) ) ;
#4023=VECTOR ( 'NONE', #12979, 1000.000000000000000 ) ;
#4063=ORIENTED_EDGE ( 'NONE', *, *, #4119, .T. ) ;
#4074=ORIENTED_EDGE ( 'NONE', *, *, #18619, .F. ) ;
#4094=VECTOR ( 'NONE', #17098, 1000.000000000000000 ) ;
#4119=EDGE_CURVE ( 'NONE', #8041, #16594, #9859, .T. ) ;
#4142=DIRECTION ( 'NONE',  ( 0.000000000000000000, 0.000000000000000000, 1.000000000000000000 ) ) ;
#4151=EDGE_CURVE ( 'NONE', #14709, #13797, #4844, .T. ) ;
#4159=CARTESIAN_POINT ( 'NONE',  ( 3.499999999999998668, -24.49999999999999289, 1.000000000000000000 ) ) ;
#4182=ORIENTED_EDGE ( 'NONE', *, *, #5534, .F. ) ;
#4194=DIRECTION ( 'NONE',  ( 0.000000000000000000, 0.000000000000000000, -1.000000000000000000 ) ) ;
#4218=LINE ( 'NONE', #7470, #8160 ) ;
#4220=DIRECTION ( 'NONE',  ( 0.000000000000000000, 0.000000000000000000, 1.000000000000000000 ) ) ;
#4235=ORIENTED_EDGE ( 'NONE', *, *, #4541, .F. ) ;
#4243=CARTESIAN_POINT ( 'NONE',  ( -14.49999999999998579, -18.49999999999999645, 4.000000000000000000 ) ) ;
#4244=DIRECTION ( 'NONE',  ( -0.000000000000000000, -0.8660254037844364872, -0.5000000000000036637 ) ) ;
#4255=ORIENTED_EDGE ( 'NONE', *, *, #9260, .T. ) ;
#4261=ORIENTED_EDGE ( 'NONE', *, *, #12949, .T. ) ;
#4282=ORIENTED_EDGE ( 'NONE', *, *, #13693, .T. ) ;
#4288=CIRCLE ( 'NONE', #12301, 1.000000000000002665 ) ;
#4305=DIRECTION ( 'NONE',  ( 0.000000000000000000, -0.8660254037844364872, -0.5000000000000036637 ) ) ;
#4342=LINE ( 'NONE', #8179, #4094 ) ;
#4376=EDGE_CURVE ( 'NONE', #9554, #3751, #13120, .T. ) ;
#4387=VECTOR ( 'NONE', #11954, 1000.000000000000000 ) ;
#4391=CARTESIAN_POINT ( 'NONE',  ( -7.500000000000000000, -25.49999999999999645, 6.500000000000000000 ) ) ;
#4395=EDGE_LOOP ( 'NONE', ( #863, #72, #15191, #3914 ) ) ;
#4406=DIRECTION ( 'NONE',  ( 0.000000000000000000, 0.000000000000000000, 1.000000000000000000 ) ) ;
#4421=ORIENTED_EDGE ( 'NONE', *, *, #14210, .F. ) ;
#4448=ORIENTED_EDGE ( 'NONE', *, *, #2388, .T. ) ;
#4451=CARTESIAN_POINT ( 'NONE',  ( -13.49999999999998401, -18.49999999999999645, 4.000000000000000000 ) ) ;
#4457=CARTESIAN_POINT ( 'NONE',  ( -3.499999999999998668, -19.50000000000000000, 1.000000000000000000 ) ) ;
#4462=AXIS2_PLACEMENT_3D ( 'NONE', #9255, #8666, #15626 ) ;
#4477=ORIENTED_EDGE ( 'NONE', *, *, #9972, .T. ) ;
#4488=ORIENTED_EDGE ( 'NONE', *, *, #15399, .F. ) ;
#4499=SHAPE_REPRESENTATION_RELATIONSHIP ( 'NONE' , 'NONE' ,  #6161, #10808 ) ;
#4508=LINE ( 'NONE', #14016, #6343 ) ;
#4541=EDGE_CURVE ( 'NONE', #13777, #1443, #1292, .T. ) ;
#4544=VERTEX_POINT ( 'NONE', #1191 ) ;
#4546=ORIENTED_EDGE ( 'NONE', *, *, #19785, .F. ) ;
#4550=LINE ( 'NONE', #9358, #12797 ) ;
#4586=CARTESIAN_POINT ( 'NONE',  ( 7.500000000000000000, -24.49999999999999289, 4.000000000000000000 ) ) ;
#4589=CARTESIAN_POINT ( 'NONE',  ( 14.50000000000001243, -25.49999999999999645, 1.000000000000000000 ) ) ;
#4590=EDGE_LOOP ( 'NONE', ( #7386, #18778, #10107, #12587 ) ) ;
#4592=VERTEX_POINT ( 'NONE', #979 ) ;
#4599=AXIS2_PLACEMENT_3D ( 'NONE', #6598, #19668, #19782 ) ;
#4609=MECHANICAL_DESIGN_GEOMETRIC_PRESENTATION_REPRESENTATION('',(#8290),#10966);
#4615=ORIENTED_EDGE ( 'NONE', *, *, #13480, .T. ) ;
#4616=CARTESIAN_POINT ( 'NONE',  ( 7.499999999999999112, -18.49999999999999645, 6.500000000000000888 ) ) ;
#4617=FACE_OUTER_BOUND ( 'NONE', #13878, .T. ) ;
#4622=VECTOR ( 'NONE', #8903, 1000.000000000000000 ) ;
#4638=VECTOR ( 'NONE', #10343, 1000.000000000000000 ) ;
#4643=ORIENTED_EDGE ( 'NONE', *, *, #13693, .F. ) ;
#4652=AXIS2_PLACEMENT_3D ( 'NONE', #6130, #1118, #13757 ) ;
#4654=FACE_OUTER_BOUND ( 'NONE', #1403, .T. ) ;
#4655=DIRECTION ( 'NONE',  ( 0.000000000000000000, 0.000000000000000000, -1.000000000000000000 ) ) ;
#4657=CARTESIAN_POINT ( 'NONE',  ( -7.499999999999999112, -19.49999999999999645, 4.000000000000000000 ) ) ;
#4683=CARTESIAN_POINT ( 'NONE',  ( -20.49999999999998224, -21.99999999999999645, 9.999999999999998224 ) ) ;
#4705=CARTESIAN_POINT ( 'NONE',  ( 11.00000000000000000, -25.49999999999999645, 4.000000000000000000 ) ) ;
#4721=VECTOR ( 'NONE', #1785, 1000.000000000000000 ) ;
#4728=AXIS2_PLACEMENT_3D ( 'NONE', #365, #6751, #5267 ) ;
#4737=AXIS2_PLACEMENT_3D ( 'NONE', #8635, #891, #15007 ) ;
#4753=CARTESIAN_POINT ( 'NONE',  ( -14.49999999999998579, -24.49999999999999289, 4.000000000000000000 ) ) ;
#4774=ORIENTED_EDGE ( 'NONE', *, *, #15250, .F. ) ;
#4775=ORIENTED_EDGE ( 'NONE', *, *, #1308, .T. ) ;
#4776=FACE_OUTER_BOUND ( 'NONE', #11745, .T. ) ;
#4806=ORIENTED_EDGE ( 'NONE', *, *, #5623, .F. ) ;
#4825=ORIENTED_EDGE ( 'NONE', *, *, #11417, .F. ) ;
#4844=LINE ( 'NONE', #14462, #7721 ) ;
#4856=EDGE_LOOP ( 'NONE', ( #18927, #4421, #1553, #14880, #11258, #15418, #2587, #11256 ) ) ;
#4860=CARTESIAN_POINT ( 'NONE',  ( 7.499999999999999112, -18.49999999999999645, 6.500000000000000888 ) ) ;
#4861=ADVANCED_FACE ( 'NONE', ( #2013, #3886 ), #16538, .T. ) ;
#4863=CARTESIAN_POINT ( 'NONE',  ( -14.49999999999998579, -21.99999999999999645, 14.18378559369222280 ) ) ;
#4878=EDGE_LOOP ( 'NONE', ( #19781, #10248 ) ) ;
#4899=ORIENTED_EDGE ( 'NONE', *, *, #566, .T. ) ;
#4904=DIRECTION ( 'NONE',  ( 1.000000000000000000, 0.000000000000000000, 0.000000000000000000 ) ) ;
#4905=ORIENTED_EDGE ( 'NONE', *, *, #2896, .F. ) ;
#4908=DIRECTION ( 'NONE',  ( -0.000000000000000000, 1.000000000000000000, -0.000000000000000000 ) ) ;
#4926=DIRECTION ( 'NONE',  ( -0.000000000000000000, 0.000000000000000000, -1.000000000000000000 ) ) ;
#4935=EDGE_CURVE ( 'NONE', #18601, #15348, #20440, .T. ) ;
#4945=CARTESIAN_POINT ( 'NONE',  ( -13.49999999999998401, -25.49999999999999645, 4.000000000000000000 ) ) ;
#4953=ORIENTED_EDGE ( 'NONE', *, *, #10552, .F. ) ;
#4961=LINE ( 'NONE', #11340, #10001 ) ;
#4974=VECTOR ( 'NONE', #10402, 1000.000000000000000 ) ;
#4988=VECTOR ( 'NONE', #11997, 1000.000000000000000 ) ;
#5005=PRODUCT_DEFINITION_SHAPE ( 'NONE', 'NONE',  #19177 ) ;
#5035=PRODUCT_DEFINITION_FORMATION_WITH_SPECIFIED_SOURCE ( 'ANY', '', #19212, .NOT_KNOWN. ) ;
#5046=DIRECTION ( 'NONE',  ( -1.000000000000000000, -0.000000000000000000, -0.000000000000000000 ) ) ;
#5068=PLANE ( 'NONE',  #14894 ) ;
#5070=VECTOR ( 'NONE', #2400, 1000.000000000000000 ) ;
#5073=CARTESIAN_POINT ( 'NONE',  ( 3.499999999999998668, -24.49999999999999289, 1.000000000000000000 ) ) ;
#5100=EDGE_CURVE ( 'NONE', #20584, #18396, #3055, .T. ) ;
#5101=( NAMED_UNIT ( * ) PLANE_ANGLE_UNIT ( ) SI_UNIT ( $, .RADIAN. ) );
#5103=FACE_OUTER_BOUND ( 'NONE', #18915, .T. ) ;
#5123=DIRECTION ( 'NONE',  ( -1.000000000000000000, 0.000000000000000000, 0.000000000000000000 ) ) ;
#5133=ORIENTED_EDGE ( 'NONE', *, *, #154, .T. ) ;
#5141=DIRECTION ( 'NONE',  ( 0.000000000000000000, 0.000000000000000000, 1.000000000000000000 ) ) ;
#5185=ORIENTED_EDGE ( 'NONE', *, *, #18702, .F. ) ;
#5193=CARTESIAN_POINT ( 'NONE',  ( 11.00000000000000000, -23.70993649053891517, 5.466506350946108483 ) ) ;
#5195=PLANE ( 'NONE',  #2988 ) ;
#5203=ORIENTED_EDGE ( 'NONE', *, *, #5657, .T. ) ;
#5209=DIRECTION ( 'NONE',  ( 0.000000000000000000, -0.000000000000000000, -1.000000000000000000 ) ) ;
#5212=EDGE_CURVE ( 'NONE', #8633, #20067, #14945, .T. ) ;
#5220=CARTESIAN_POINT ( 'NONE',  ( 13.49999999999998401, -21.99999999999999645, 11.68378559369222280 ) ) ;
#5230=ORIENTED_EDGE ( 'NONE', *, *, #82, .F. ) ;
#5233=CARTESIAN_POINT ( 'NONE',  ( 20.49999999999998224, -21.99999999999999645, 12.00000000000000355 ) ) ;
#5237=CARTESIAN_POINT ( 'NONE',  ( 11.00000000000000000, -19.49999999999999645, 4.000000000000000000 ) ) ;
#5246=CARTESIAN_POINT ( 'NONE',  ( 0.000000000000000000, 0.000000000000000000, 4.000000000000000000 ) ) ;
#5257=LINE ( 'NONE', #12895, #20713 ) ;
#5258=ORIENTED_EDGE ( 'NONE', *, *, #14014, .F. ) ;
#5267=DIRECTION ( 'NONE',  ( 0.000000000000000000, 0.000000000000000000, -1.000000000000000000 ) ) ;
#5272=DIRECTION ( 'NONE',  ( 0.000000000000000000, 0.000000000000000000, 1.000000000000000000 ) ) ;
#5304=ORIENTED_EDGE ( 'NONE', *, *, #18166, .F. ) ;
#5308=CARTESIAN_POINT ( 'NONE',  ( -7.500000000000000000, -23.70993649053891517, 5.466506350946108483 ) ) ;
#5317=FACE_OUTER_BOUND ( 'NONE', #10934, .T. ) ;
#5318=ADVANCED_FACE ( 'NONE', ( #19783 ), #3556, .F. ) ;
#5324=DIRECTION ( 'NONE',  ( 1.000000000000000000, 0.000000000000000000, 0.000000000000000000 ) ) ;
#5326=CARTESIAN_POINT ( 'NONE',  ( 7.499999999999999112, -18.49999999999999645, 4.000000000000000000 ) ) ;
#5337=FACE_OUTER_BOUND ( 'NONE', #8410, .T. ) ;
#5343=ORIENTED_EDGE ( 'NONE', *, *, #19264, .F. ) ;
#5351=VECTOR ( 'NONE', #9846, 1000.000000000000000 ) ;
#5355=DIRECTION ( 'NONE',  ( 0.000000000000000000, 0.000000000000000000, 1.000000000000000000 ) ) ;
#5372=CIRCLE ( 'NONE', #4728, 0.2500000000000002220 ) ;
#5400=ORIENTED_EDGE ( 'NONE', *, *, #9108, .T. ) ;
#5414=ORIENTED_EDGE ( 'NONE', *, *, #19382, .T. ) ;
#5424=DIRECTION ( 'NONE',  ( 0.000000000000000000, 0.000000000000000000, 1.000000000000000000 ) ) ;
#5426=ADVANCED_FACE ( 'NONE', ( #5856 ), #19982, .T. ) ;
#5440=EDGE_CURVE ( 'NONE', #3175, #3061, #10560, .T. ) ;
#5449=DIRECTION ( 'NONE',  ( -0.000000000000000000, -0.000000000000000000, -1.000000000000000000 ) ) ;
#5458=CIRCLE ( 'NONE', #6469, 0.2500000000000002220 ) ;
#5474=LINE ( 'NONE', #16649, #7106 ) ;
#5486=ORIENTED_EDGE ( 'NONE', *, *, #2703, .F. ) ;
#5501=EDGE_CURVE ( 'NONE', #3437, #20223, #9193, .T. ) ;
#5502=FACE_OUTER_BOUND ( 'NONE', #9143, .T. ) ;
#5521=CIRCLE ( 'NONE', #10495, 2.500000000000000444 ) ;
#5528=ADVANCED_FACE ( 'NONE', ( #20196 ), #13484, .F. ) ;
#5530=LINE ( 'NONE', #20080, #15376 ) ;
#5531=FACE_OUTER_BOUND ( 'NONE', #16567, .T. ) ;
#5534=EDGE_CURVE ( 'NONE', #13135, #13151, #10353, .T. ) ;
#5544=DIRECTION ( 'NONE',  ( 0.000000000000000000, 0.000000000000000000, -1.000000000000000000 ) ) ;
#5548=DIRECTION ( 'NONE',  ( 0.000000000000000000, 0.8660254037844363761, -0.5000000000000041078 ) ) ;
#5549=SURFACE_SIDE_STYLE ('',( #13493 ) ) ;
#5551=CARTESIAN_POINT ( 'NONE',  ( -2.499999999999998224, -24.49999999999999289, 1.000000000000000000 ) ) ;
#5574=LINE ( 'NONE', #8417, #9773 ) ;
#5595=ORIENTED_EDGE ( 'NONE', *, *, #7459, .T. ) ;
#5603=ORIENTED_EDGE ( 'NONE', *, *, #1709, .T. ) ;
#5618=ORIENTED_EDGE ( 'NONE', *, *, #19739, .T. ) ;
#5623=EDGE_CURVE ( 'NONE', #8041, #3395, #20510, .T. ) ;
#5626=ORIENTED_EDGE ( 'NONE', *, *, #10789, .T. ) ;
#5634=FACE_BOUND ( 'NONE', #13608, .T. ) ;
#5645=VECTOR ( 'NONE', #16685, 1000.000000000000000 ) ;
#5649=AXIS2_PLACEMENT_3D ( 'NONE', #16298, #3231, #5209 ) ;
#5657=EDGE_CURVE ( 'NONE', #8747, #11334, #17551, .T. ) ;
#5658=EDGE_CURVE ( 'NONE', #6686, #18235, #2919, .T. ) ;
#5663=CARTESIAN_POINT ( 'NONE',  ( -13.49999999999998401, -18.49999999999999645, 4.000000000000000000 ) ) ;
#5682=VERTEX_POINT ( 'NONE', #9296 ) ;
#5688=LINE ( 'NONE', #15505, #13056 ) ;
#5715=DIRECTION ( 'NONE',  ( 0.000000000000000000, -1.000000000000000000, 0.000000000000000000 ) ) ;
#5719=VECTOR ( 'NONE', #19388, 1000.000000000000000 ) ;
#5722=LINE ( 'NONE', #1120, #2512 ) ;
#5737=FACE_OUTER_BOUND ( 'NONE', #16733, .T. ) ;
#5758=PLANE ( 'NONE',  #8322 ) ;
#5760=ORIENTED_EDGE ( 'NONE', *, *, #15250, .T. ) ;
#5808=ORIENTED_EDGE ( 'NONE', *, *, #15862, .F. ) ;
#5816=VERTEX_POINT ( 'NONE', #2393 ) ;
#5821=CARTESIAN_POINT ( 'NONE',  ( 7.499999999999999112, -18.49999999999999645, 6.500000000000000888 ) ) ;
#5826=CARTESIAN_POINT ( 'NONE',  ( 11.00000000000000000, -25.49999999999999645, 6.500000000000000000 ) ) ;
#5829=DIRECTION ( 'NONE',  ( 0.000000000000000000, -0.000000000000000000, -1.000000000000000000 ) ) ;
#5844=CARTESIAN_POINT ( 'NONE',  ( -14.49999999999998579, -24.49999999999999289, 4.000000000000000000 ) ) ;
#5856=FACE_OUTER_BOUND ( 'NONE', #3698, .T. ) ;
#5887=DIRECTION ( 'NONE',  ( 0.000000000000000000, 0.000000000000000000, 1.000000000000000000 ) ) ;
#5893=CARTESIAN_POINT ( 'NONE',  ( -11.00000000000000000, -20.16506350946107418, 5.250000000000000000 ) ) ;
#5898=VERTEX_POINT ( 'NONE', #6445 ) ;
#5900=FACE_OUTER_BOUND ( 'NONE', #9664, .T. ) ;
#5903=VERTEX_POINT ( 'NONE', #2992 ) ;
#5907=ORIENTED_EDGE ( 'NONE', *, *, #14210, .T. ) ;
#5908=CARTESIAN_POINT ( 'NONE',  ( 13.50000000000001243, -19.49999999999999645, 1.000000000000000000 ) ) ;
#5914=EDGE_CURVE ( 'NONE', #15986, #2296, #19415, .T. ) ;
#5932=ORIENTED_EDGE ( 'NONE', *, *, #12798, .T. ) ;
#5938=ORIENTED_EDGE ( 'NONE', *, *, #281, .T. ) ;
#5951=DIRECTION ( 'NONE',  ( 0.000000000000000000, 0.000000000000000000, -1.000000000000000000 ) ) ;
#5955=EDGE_CURVE ( 'NONE', #1443, #20090, #14264, .T. ) ;
#5966=VERTEX_POINT ( 'NONE', #16058 ) ;
#5975=AXIS2_PLACEMENT_3D ( 'NONE', #12728, #3315, #14089 ) ;
#6005=PLANE ( 'NONE',  #8390 ) ;
#6052=LINE ( 'NONE', #14088, #3976 ) ;
#6065=DIRECTION ( 'NONE',  ( 0.000000000000000000, 0.1264857625231113059, -0.9919684228235025047 ) ) ;
#6081=CARTESIAN_POINT ( 'NONE',  ( 11.00000000000000000, -20.16506350946107418, 5.250000000000000000 ) ) ;
#6113=CARTESIAN_POINT ( 'NONE',  ( 7.499999999999999112, -23.70993649053891517, 5.466506350946108483 ) ) ;
#6130=CARTESIAN_POINT ( 'NONE',  ( -20.49999999999998224, -21.99999999999999645, 11.00000000000000178 ) ) ;
#6161=SHAPE_REPRESENTATION ( 'spring housing', ( #18039 ), #15032 ) ;
#6164=CARTESIAN_POINT ( 'NONE',  ( 11.00000000000000000, -20.29006350946107418, 5.466506350946110260 ) ) ;
#6170=EDGE_LOOP ( 'NONE', ( #1413, #18671, #4643, #13388, #3461, #19865, #5808, #7585, #14855, #14050, #2585, #8182 ) ) ;
#6193=ORIENTED_EDGE ( 'NONE', *, *, #11641, .F. ) ;
#6196=AXIS2_PLACEMENT_3D ( 'NONE', #13045, #17862, #1960 ) ;
#6240=PLANE ( 'NONE',  #15650 ) ;
#6265=FACE_OUTER_BOUND ( 'NONE', #2865, .T. ) ;
#6280=LINE ( 'NONE', #1575, #16397 ) ;
#6295=CIRCLE ( 'NONE', #2623, 0.2500000000000002220 ) ;
#6319=VECTOR ( 'NONE', #5544, 1000.000000000000000 ) ;
#6335=LINE ( 'NONE', #11453, #10650 ) ;
#6343=VECTOR ( 'NONE', #16112, 1000.000000000000000 ) ;
#6364=( LENGTH_UNIT ( ) NAMED_UNIT ( * ) SI_UNIT ( .MILLI., .METRE. ) );
#6378=EDGE_LOOP ( 'NONE', ( #16151, #12002, #12511, #4448 ) ) ;
#6380=( LENGTH_UNIT ( ) NAMED_UNIT ( * ) SI_UNIT ( .MILLI., .METRE. ) );
#6403=CIRCLE ( 'NONE', #4599, 1.000000000000002665 ) ;
#6411=CARTESIAN_POINT ( 'NONE',  ( 13.49999999999998401, -24.47992105705875332, 12.00000000000000000 ) ) ;
#6433=EDGE_LOOP ( 'NONE', ( #19141, #15004, #18087, #17264, #12137, #17651 ) ) ;
#6445=CARTESIAN_POINT ( 'NONE',  ( 3.499999999999999556, -24.49999999999999289, 4.000000000000000000 ) ) ;
#6447=DIRECTION ( 'NONE',  ( 0.000000000000000000, -0.9919684228235026158, -0.1264857625231113336 ) ) ;
#6460=DIRECTION ( 'NONE',  ( -0.000000000000000000, 0.000000000000000000, 1.000000000000000000 ) ) ;
#6467=ORIENTED_EDGE ( 'NONE', *, *, #795, .F. ) ;
#6469=AXIS2_PLACEMENT_3D ( 'NONE', #332, #1160, #2613 ) ;
#6507=VERTEX_POINT ( 'NONE', #12695 ) ;
#6513=CARTESIAN_POINT ( 'NONE',  ( -14.49999999999998579, -21.99999999999999645, 11.00000000000000178 ) ) ;
#6520=FACE_OUTER_BOUND ( 'NONE', #11253, .T. ) ;
#6524=ORIENTED_EDGE ( 'NONE', *, *, #15761, .F. ) ;
#6538=FACE_OUTER_BOUND ( 'NONE', #20518, .T. ) ;
#6540=DIRECTION ( 'NONE',  ( -1.000000000000000000, -1.734723475976809067E-16, 0.000000000000000000 ) ) ;
#6558=ORIENTED_EDGE ( 'NONE', *, *, #19357, .T. ) ;
#6562=VERTEX_POINT ( 'NONE', #1724 ) ;
#6564=DIRECTION ( 'NONE',  ( 0.000000000000000000, 0.000000000000000000, 1.000000000000000000 ) ) ;
#6569=DIRECTION ( 'NONE',  ( -1.000000000000000000, -0.000000000000000000, -0.000000000000000000 ) ) ;
#6598=CARTESIAN_POINT ( 'NONE',  ( 14.49999999999998579, -21.99999999999999645, 11.00000000000000178 ) ) ;
#6632=CARTESIAN_POINT ( 'NONE',  ( 14.49999999999998579, -21.99999999999999645, 9.999999999999998224 ) ) ;
#6637=FACE_OUTER_BOUND ( 'NONE', #12481, .T. ) ;
#6672=SURFACE_STYLE_USAGE ( .BOTH. , #1958 ) ;
#6685=VECTOR ( 'NONE', #10490, 1000.000000000000000 ) ;
#6686=VERTEX_POINT ( 'NONE', #11542 ) ;
#6689=AXIS2_PLACEMENT_3D ( 'NONE', #5220, #14533, #17783 ) ;
#6694=EDGE_CURVE ( 'NONE', #8351, #2802, #5474, .T. ) ;
#6748=AXIS2_PLACEMENT_3D ( 'NONE', #18722, #3965, #2602 ) ;
#6751=DIRECTION ( 'NONE',  ( 1.000000000000000000, -0.000000000000000000, -0.000000000000000000 ) ) ;
#6788=PLANE ( 'NONE',  #5649 ) ;
#6810=ORIENTED_EDGE ( 'NONE', *, *, #82, .T. ) ;
#6829=EDGE_CURVE ( 'NONE', #3840, #11512, #5574, .T. ) ;
#6837=VERTEX_POINT ( 'NONE', #13207 ) ;
#6871=FACE_OUTER_BOUND ( 'NONE', #14204, .T. ) ;
#6878=ORIENTED_EDGE ( 'NONE', *, *, #9108, .F. ) ;
#6886=PRODUCT_CONTEXT ( 'NONE', #7340, 'mechanical' ) ;
#6904=LINE ( 'NONE', #16521, #6319 ) ;
#6911=CARTESIAN_POINT ( 'NONE',  ( -13.49999999999998401, -25.49999999999999645, 4.000000000000000000 ) ) ;
#6928=ADVANCED_FACE ( 'NONE', ( #8921 ), #17073, .T. ) ;
#6935=EDGE_LOOP ( 'NONE', ( #13465, #13971, #19757, #1107 ) ) ;
#6956=EDGE_LOOP ( 'NONE', ( #3180, #10242, #1836, #4282, #9720, #7102 ) ) ;
#6974=VECTOR ( 'NONE', #16486, 1000.000000000000000 ) ;
#6992=VECTOR ( 'NONE', #15533, 1000.000000000000000 ) ;
#7014=VECTOR ( 'NONE', #8674, 1000.000000000000000 ) ;
#7071=ORIENTED_EDGE ( 'NONE', *, *, #12449, .F. ) ;
#7080=ORIENTED_EDGE ( 'NONE', *, *, #11417, .T. ) ;
#7102=ORIENTED_EDGE ( 'NONE', *, *, #8015, .F. ) ;
#7106=VECTOR ( 'NONE', #4007, 1000.000000000000000 ) ;
#7110=CARTESIAN_POINT ( 'NONE',  ( 2.499999999999998668, -19.50000000000000000, 1.000000000000000000 ) ) ;
#7111=EDGE_CURVE ( 'NONE', #18396, #814, #1771, .T. ) ;
#7125=ORIENTED_EDGE ( 'NONE', *, *, #1030, .T. ) ;
#7129=LINE ( 'NONE', #13492, #16778 ) ;
#7130=FILL_AREA_STYLE ('',( #3978 ) ) ;
#7131=ORIENTED_EDGE ( 'NONE', *, *, #12824, .F. ) ;
#7139=CARTESIAN_POINT ( 'NONE',  ( 11.00000000000000000, -23.83493649053891517, 4.999999999999999112 ) ) ;
#7148=VECTOR ( 'NONE', #1998, 1000.000000000000000 ) ;
#7149=EDGE_LOOP ( 'NONE', ( #9718, #19248, #15719, #5595, #14497, #4825 ) ) ;
#7154=EDGE_LOOP ( 'NONE', ( #5230, #17777, #3541, #7748 ) ) ;
#7157=DIRECTION ( 'NONE',  ( -0.000000000000000000, -0.8660254037844363761, 0.5000000000000041078 ) ) ;
#7176=ORIENTED_EDGE ( 'NONE', *, *, #10552, .T. ) ;
#7178=VERTEX_POINT ( 'NONE', #3163 ) ;
#7180=VERTEX_POINT ( 'NONE', #12663 ) ;
#7211=ADVANCED_FACE ( 'NONE', ( #12563 ), #15706, .F. ) ;
#7212=PLANE ( 'NONE',  #3016 ) ;
#7252=ORIENTED_EDGE ( 'NONE', *, *, #2362, .T. ) ;
#7256=LINE ( 'NONE', #8829, #7966 ) ;
#7266=VECTOR ( 'NONE', #19148, 1000.000000000000227 ) ;
#7271=ORIENTED_EDGE ( 'NONE', *, *, #19739, .F. ) ;
#7275=ORIENTED_EDGE ( 'NONE', *, *, #2171, .T. ) ;
#7297=ORIENTED_EDGE ( 'NONE', *, *, #12365, .T. ) ;
#7310=LINE ( 'NONE', #16920, #4638 ) ;
#7313=VECTOR ( 'NONE', #19970, 1000.000000000000000 ) ;
#7314=CARTESIAN_POINT ( 'NONE',  ( 11.00000000000000000, -20.29006350946107418, 5.466506350946110260 ) ) ;
#7320=DIRECTION ( 'NONE',  ( 0.000000000000000000, 0.000000000000000000, 1.000000000000000000 ) ) ;
#7340=APPLICATION_CONTEXT ( 'automotive_design' ) ;
#7364=DIRECTION ( 'NONE',  ( 1.000000000000000000, -0.000000000000000000, 0.000000000000000000 ) ) ;
#7366=FACE_OUTER_BOUND ( 'NONE', #2825, .T. ) ;
#7368=ADVANCED_FACE ( 'NONE', ( #19486 ), #10054, .T. ) ;
#7379=VERTEX_POINT ( 'NONE', #6911 ) ;
#7386=ORIENTED_EDGE ( 'NONE', *, *, #3038, .F. ) ;
#7402=CARTESIAN_POINT ( 'NONE',  ( -14.49999999999998579, -25.49999999999999645, 1.000000000000000000 ) ) ;
#7416=VERTEX_POINT ( 'NONE', #14759 ) ;
#7428=EDGE_LOOP ( 'NONE', ( #17152, #4905, #10208, #5618 ) ) ;
#7430=DIRECTION ( 'NONE',  ( -1.000000000000000000, -0.000000000000000000, -0.000000000000000000 ) ) ;
#7459=EDGE_CURVE ( 'NONE', #7178, #8633, #5458, .T. ) ;
#7462=VERTEX_POINT ( 'NONE', #5551 ) ;
#7468=DIRECTION ( 'NONE',  ( 0.000000000000000000, 0.1264857625231113059, 0.9919684228235025047 ) ) ;
#7470=CARTESIAN_POINT ( 'NONE',  ( 11.00000000000000000, -20.16506350946107418, 5.000000000000000000 ) ) ;
#7520=CARTESIAN_POINT ( 'NONE',  ( 2.499999999999999112, -24.49999999999999289, 4.000000000000000000 ) ) ;
#7568=DIRECTION ( 'NONE',  ( 1.000000000000000000, 0.000000000000000000, 0.000000000000000000 ) ) ;
#7570=CARTESIAN_POINT ( 'NONE',  ( 11.00000000000000000, -24.49999999999999289, 5.000000000000000000 ) ) ;
#7581=LINE ( 'NONE', #17196, #11063 ) ;
#7585=ORIENTED_EDGE ( 'NONE', *, *, #12949, .F. ) ;
#7589=ORIENTED_EDGE ( 'NONE', *, *, #9972, .F. ) ;
#7591=DIRECTION ( 'NONE',  ( -1.000000000000000000, -0.000000000000000000, -0.000000000000000000 ) ) ;
#7607=LINE ( 'NONE', #17123, #10970 ) ;
#7621=VECTOR ( 'NONE', #13462, 1000.000000000000000 ) ;
#7629=PLANE ( 'NONE',  #10668 ) ;
#7656=ORIENTED_EDGE ( 'NONE', *, *, #3038, .T. ) ;
#7670=CARTESIAN_POINT ( 'NONE',  ( 11.00000000000000000, -23.83493649053891517, 4.999999999999999112 ) ) ;
#7677=DIRECTION ( 'NONE',  ( 0.000000000000000000, 0.000000000000000000, 1.000000000000000000 ) ) ;
#7678=EDGE_CURVE ( 'NONE', #14333, #11513, #12456, .T. ) ;
#7681=AXIS2_PLACEMENT_3D ( 'NONE', #7958, #14332, #9326 ) ;
#7696=STYLED_ITEM ( 'NONE', ( #15168 ), #10808 ) ;
#7702=DIRECTION ( 'NONE',  ( -1.000000000000000000, -0.000000000000000000, -0.000000000000000000 ) ) ;
#7708=EDGE_CURVE ( 'NONE', #7379, #5682, #14419, .T. ) ;
#7713=EDGE_LOOP ( 'NONE', ( #9390, #403, #12156, #10098 ) ) ;
#7714=CARTESIAN_POINT ( 'NONE',  ( -7.499999999999999112, -24.49999999999999289, 4.000000000000000000 ) ) ;
#7721=VECTOR ( 'NONE', #1912, 1000.000000000000000 ) ;
#7745=LINE ( 'NONE', #18935, #7266 ) ;
#7748=ORIENTED_EDGE ( 'NONE', *, *, #6694, .T. ) ;
#7754=LINE ( 'NONE', #20425, #2330 ) ;
#7772=DIRECTION ( 'NONE',  ( -0.000000000000000000, 0.000000000000000000, -1.000000000000000000 ) ) ;
#7777=AXIS2_PLACEMENT_3D ( 'NONE', #6513, #1698, #7866 ) ;
#7790=ORIENTED_EDGE ( 'NONE', *, *, #8472, .F. ) ;
#7816=CARTESIAN_POINT ( 'NONE',  ( -7.499999999999999112, -19.49999999999999645, 4.000000000000000000 ) ) ;
#7824=EDGE_CURVE ( 'NONE', #2297, #10229, #103, .T. ) ;
#7826=CARTESIAN_POINT ( 'NONE',  ( 11.00000000000000000, -24.49999999999999289, 4.000000000000000000 ) ) ;
#7829=EDGE_CURVE ( 'NONE', #8633, #10619, #15683, .T. ) ;
#7840=ORIENTED_EDGE ( 'NONE', *, *, #19877, .F. ) ;
#7851=DIRECTION ( 'NONE',  ( 8.673617379884047798E-17, -1.000000000000000000, 0.000000000000000000 ) ) ;
#7856=DIRECTION ( 'NONE',  ( 1.000000000000000000, -0.000000000000000000, -0.000000000000000000 ) ) ;
#7866=DIRECTION ( 'NONE',  ( 0.000000000000000000, 0.000000000000000000, 1.000000000000000000 ) ) ;
#7891=ORIENTED_EDGE ( 'NONE', *, *, #566, .F. ) ;
#7952=EDGE_CURVE ( 'NONE', #20223, #18461, #13363, .T. ) ;
#7958=CARTESIAN_POINT ( 'NONE',  ( -14.49999999999998579, -19.49999999999999645, 4.000000000000000000 ) ) ;
#7966=VECTOR ( 'NONE', #7157, 1000.000000000000000 ) ;
#7969=DIRECTION ( 'NONE',  ( -1.000000000000000000, 0.000000000000000000, 0.000000000000000000 ) ) ;
#7971=CARTESIAN_POINT ( 'NONE',  ( 14.50000000000001243, -25.49999999999999645, 4.000000000000000000 ) ) ;
#7984=ADVANCED_FACE ( 'NONE', ( #5317 ), #3544, .T. ) ;
#7999=CARTESIAN_POINT ( 'NONE',  ( -3.499999999999998668, -19.50000000000000000, 1.000000000000000000 ) ) ;
#8015=EDGE_CURVE ( 'NONE', #3751, #11612, #4550, .T. ) ;
#8018=EDGE_LOOP ( 'NONE', ( #17769, #3324, #18934, #10828, #6193, #4235, #14439, #5907 ) ) ;
#8020=DIRECTION ( 'NONE',  ( -0.000000000000000000, 0.000000000000000000, -1.000000000000000000 ) ) ;
#8035=SURFACE_STYLE_FILL_AREA ( #185 ) ;
#8041=VERTEX_POINT ( 'NONE', #1212 ) ;
#8043=CARTESIAN_POINT ( 'NONE',  ( 13.49999999999998401, -18.49999999999999645, 4.000000000000000000 ) ) ;
#8055=CARTESIAN_POINT ( 'NONE',  ( -14.49999999999998579, -25.49999999999999645, 4.000000000000000000 ) ) ;
#8062=VECTOR ( 'NONE', #19717, 1000.000000000000000 ) ;
#8079=ORIENTED_EDGE ( 'NONE', *, *, #281, .F. ) ;
#8080=AXIS2_PLACEMENT_3D ( 'NONE', #18204, #16611, #736 ) ;
#8095=ADVANCED_FACE ( 'NONE', ( #17410 ), #17202, .T. ) ;
#8112=DIRECTION ( 'NONE',  ( 1.000000000000000000, 0.000000000000000000, -0.000000000000000000 ) ) ;
#8116=CARTESIAN_POINT ( 'NONE',  ( 20.49999999999998224, -21.99999999999999645, 12.00000000000000355 ) ) ;
#8160=VECTOR ( 'NONE', #11953, 1000.000000000000000 ) ;
#8167=CYLINDRICAL_SURFACE ( 'NONE', #6689, 2.500000000000000444 ) ;
#8179=CARTESIAN_POINT ( 'NONE',  ( 14.50000000000001243, -18.49999999999999645, 4.000000000000000000 ) ) ;
#8180=DIRECTION ( 'NONE',  ( 1.000000000000000000, 0.000000000000000000, 0.000000000000000000 ) ) ;
#8182=ORIENTED_EDGE ( 'NONE', *, *, #9182, .F. ) ;
#8206=ADVANCED_FACE ( 'NONE', ( #17613 ), #9872, .T. ) ;
#8210=ADVANCED_FACE ( 'NONE', ( #6637 ), #5068, .T. ) ;
#8215=DIRECTION ( 'NONE',  ( 0.000000000000000000, 0.000000000000000000, -1.000000000000000000 ) ) ;
#8225=VERTEX_POINT ( 'NONE', #3494 ) ;
#8237=CARTESIAN_POINT ( 'NONE',  ( -11.00000000000000000, -20.29006350946107418, 5.466506350946110260 ) ) ;
#8249=VECTOR ( 'NONE', #13209, 1000.000000000000000 ) ;
#8252=LINE ( 'NONE', #11277, #10997 ) ;
#8273=ADVANCED_FACE ( 'NONE', ( #6538 ), #1923, .T. ) ;
#8280=LINE ( 'NONE', #16233, #5351 ) ;
#8290=STYLED_ITEM ( 'NONE', ( #11480 ), #17970 ) ;
#8305=DIRECTION ( 'NONE',  ( -1.000000000000000000, -8.673617379884045333E-17, 0.000000000000000000 ) ) ;
#8306=AXIS2_PLACEMENT_3D ( 'NONE', #13017, #6447, #11243 ) ;
#8322=AXIS2_PLACEMENT_3D ( 'NONE', #16731, #10565, #16933 ) ;
#8325=CARTESIAN_POINT ( 'NONE',  ( 7.499999999999999112, -25.49999999999999645, 6.500000000000000888 ) ) ;
#8351=VERTEX_POINT ( 'NONE', #10394 ) ;
#8354=DIRECTION ( 'NONE',  ( 0.000000000000000000, 0.000000000000000000, 1.000000000000000000 ) ) ;
#8355=MECHANICAL_DESIGN_GEOMETRIC_PRESENTATION_REPRESENTATION('',(#7696),#11363);
#8364=VECTOR ( 'NONE', #13931, 1000.000000000000000 ) ;
#8383=CARTESIAN_POINT ( 'NONE',  ( 13.50000000000001243, -24.49999999999999289, 4.000000000000000000 ) ) ;
#8385=ORIENTED_EDGE ( 'NONE', *, *, #11684, .F. ) ;
#8390=AXIS2_PLACEMENT_3D ( 'NONE', #4945, #11027, #3078 ) ;
#8410=EDGE_LOOP ( 'NONE', ( #7275, #15493, #13821, #7071 ) ) ;
#8417=CARTESIAN_POINT ( 'NONE',  ( 13.49999999999998401, -18.49999999999999645, 4.000000000000000000 ) ) ;
#8418=CARTESIAN_POINT ( 'NONE',  ( 3.499999999999998668, -19.50000000000000000, 1.000000000000000000 ) ) ;
#8426=LINE ( 'NONE', #11956, #2680 ) ;
#8472=EDGE_CURVE ( 'NONE', #15081, #20661, #2029, .T. ) ;
#8493=LINE ( 'NONE', #12141, #842 ) ;
#8509=ADVANCED_FACE ( 'NONE', ( #18031 ), #2130, .T. ) ;
#8538=ORIENTED_EDGE ( 'NONE', *, *, #528, .F. ) ;
#8557=ORIENTED_EDGE ( 'NONE', *, *, #293, .T. ) ;
#8590=DIRECTION ( 'NONE',  ( 0.000000000000000000, 0.000000000000000000, -1.000000000000000000 ) ) ;
#8612=ADVANCED_FACE ( 'NONE', ( #4617 ), #3261, .T. ) ;
#8626=VERTEX_POINT ( 'NONE', #6411 ) ;
#8633=VERTEX_POINT ( 'NONE', #12775 ) ;
#8635=CARTESIAN_POINT ( 'NONE',  ( 14.50000000000001243, -18.49999999999999645, 4.000000000000000000 ) ) ;
#8666=DIRECTION ( 'NONE',  ( 0.000000000000000000, 1.000000000000000000, -0.000000000000000000 ) ) ;
#8674=DIRECTION ( 'NONE',  ( -1.000000000000000000, -0.000000000000000000, -0.000000000000000000 ) ) ;
#8688=EDGE_LOOP ( 'NONE', ( #6878, #14851, #18908, #1505, #8899, #14726, #14445, #8965 ) ) ;
#8700=LINE ( 'NONE', #7139, #9063 ) ;
#8717=VECTOR ( 'NONE', #7468, 1000.000000000000227 ) ;
#8736=ORIENTED_EDGE ( 'NONE', *, *, #19153, .T. ) ;
#8744=ORIENTED_EDGE ( 'NONE', *, *, #12700, .F. ) ;
#8747=VERTEX_POINT ( 'NONE', #948 ) ;
#8782=DIRECTION ( 'NONE',  ( -0.000000000000000000, 0.000000000000000000, 1.000000000000000000 ) ) ;
#8789=ORIENTED_EDGE ( 'NONE', *, *, #10380, .F. ) ;
#8795=DIRECTION ( 'NONE',  ( 0.000000000000000000, 0.000000000000000000, -1.000000000000000000 ) ) ;
#8800=SURFACE_STYLE_USAGE ( .BOTH. , #5549 ) ;
#8819=ORIENTED_EDGE ( 'NONE', *, *, #20608, .F. ) ;
#8822=LINE ( 'NONE', #2430, #6685 ) ;
#8829=CARTESIAN_POINT ( 'NONE',  ( 11.00000000000000000, -25.49999999999999645, 6.500000000000000000 ) ) ;
#8846=ORIENTED_EDGE ( 'NONE', *, *, #20468, .T. ) ;
#8848=DIRECTION ( 'NONE',  ( -1.000000000000000000, 0.000000000000000000, 0.000000000000000000 ) ) ;
#8862=PLANE ( 'NONE',  #15225 ) ;
#8878=CARTESIAN_POINT ( 'NONE',  ( -14.49999999999998579, -18.49999999999999645, 4.000000000000000000 ) ) ;
#8880=DIRECTION ( 'NONE',  ( -0.000000000000000000, -0.000000000000000000, -1.000000000000000000 ) ) ;
#8899=ORIENTED_EDGE ( 'NONE', *, *, #10162, .T. ) ;
#8902=EDGE_CURVE ( 'NONE', #95, #15413, #20619, .T. ) ;
#8903=DIRECTION ( 'NONE',  ( 1.000000000000000000, -0.000000000000000000, 0.000000000000000000 ) ) ;
#8921=FACE_OUTER_BOUND ( 'NONE', #4878, .T. ) ;
#8965=ORIENTED_EDGE ( 'NONE', *, *, #9182, .T. ) ;
#8975=LINE ( 'NONE', #5844, #625 ) ;
#8981=VECTOR ( 'NONE', #12609, 1000.000000000000000 ) ;
#8990=AXIS2_PLACEMENT_3D ( 'NONE', #9590, #20285, #12524 ) ;
#8995=FACE_OUTER_BOUND ( 'NONE', #13626, .T. ) ;
#9038=CARTESIAN_POINT ( 'NONE',  ( -14.49999999999998579, -18.49999999999999645, 4.000000000000000000 ) ) ;
#9063=VECTOR ( 'NONE', #5046, 1000.000000000000000 ) ;
#9069=LINE ( 'NONE', #13964, #19042 ) ;
#9078=VERTEX_POINT ( 'NONE', #8878 ) ;
#9098=EDGE_CURVE ( 'NONE', #12874, #16270, #20390, .T. ) ;
#9102=EDGE_LOOP ( 'NONE', ( #1463, #3206 ) ) ;
#9108=EDGE_CURVE ( 'NONE', #13797, #14476, #12314, .T. ) ;
#9130=CARTESIAN_POINT ( 'NONE',  ( 20.49999999999998224, -21.99999999999999645, 11.00000000000000178 ) ) ;
#9143=EDGE_LOOP ( 'NONE', ( #2250, #4615, #292, #17691 ) ) ;
#9145=FACE_OUTER_BOUND ( 'NONE', #7154, .T. ) ;
#9153=ORIENTED_EDGE ( 'NONE', *, *, #9098, .T. ) ;
#9160=LINE ( 'NONE', #1214, #15960 ) ;
#9161=PLANE ( 'NONE',  #315 ) ;
#9182=EDGE_CURVE ( 'NONE', #95, #14476, #8975, .T. ) ;
#9183=DIRECTION ( 'NONE',  ( 0.000000000000000000, 0.000000000000000000, 1.000000000000000000 ) ) ;
#9186=LINE ( 'NONE', #1243, #9383 ) ;
#9193=LINE ( 'NONE', #20294, #14083 ) ;
#9195=VERTEX_POINT ( 'NONE', #12215 ) ;
#9213=CARTESIAN_POINT ( 'NONE',  ( -13.49999999999998401, -18.49999999999999645, 1.000000000000000000 ) ) ;
#9224=DIRECTION ( 'NONE',  ( 0.000000000000000000, 0.000000000000000000, -1.000000000000000000 ) ) ;
#9255=CARTESIAN_POINT ( 'NONE',  ( -14.49999999999998579, -24.49999999999999289, 4.000000000000000000 ) ) ;
#9260=EDGE_CURVE ( 'NONE', #14806, #20584, #3296, .T. ) ;
#9265=CARTESIAN_POINT ( 'NONE',  ( 14.49999999999998579, -21.99999999999999645, 11.00000000000000178 ) ) ;
#9274=CARTESIAN_POINT ( 'NONE',  ( -14.49999999999998579, -24.49999999999999289, 1.000000000000000000 ) ) ;
#9281=CARTESIAN_POINT ( 'NONE',  ( 3.499999999999998668, -19.50000000000000000, 1.000000000000000000 ) ) ;
#9296=CARTESIAN_POINT ( 'NONE',  ( -11.00000000000000000, -25.49999999999999645, 4.000000000000000000 ) ) ;
#9319=VECTOR ( 'NONE', #16834, 1000.000000000000000 ) ;
#9326=DIRECTION ( 'NONE',  ( 0.000000000000000000, -0.000000000000000000, -1.000000000000000000 ) ) ;
#9358=CARTESIAN_POINT ( 'NONE',  ( 7.499999999999999112, -25.49999999999999645, 6.500000000000000000 ) ) ;
#9360=VECTOR ( 'NONE', #8880, 1000.000000000000000 ) ;
#9363=CARTESIAN_POINT ( 'NONE',  ( -13.49999999999998401, -21.99999999999999645, 11.68378559369222280 ) ) ;
#9367=PLANE ( 'NONE',  #19228 ) ;
#9370=LINE ( 'NONE', #2569, #15661 ) ;
#9383=VECTOR ( 'NONE', #9395, 1000.000000000000000 ) ;
#9390=ORIENTED_EDGE ( 'NONE', *, *, #11641, .T. ) ;
#9395=DIRECTION ( 'NONE',  ( 1.000000000000000000, 0.000000000000000000, 0.000000000000000000 ) ) ;
#9407=DIRECTION ( 'NONE',  ( 1.000000000000000000, 0.000000000000000000, 0.000000000000000000 ) ) ;
#9414=EDGE_CURVE ( 'NONE', #10619, #12385, #14814, .T. ) ;
#9416=VERTEX_POINT ( 'NONE', #16382 ) ;
#9489=ORIENTED_EDGE ( 'NONE', *, *, #4119, .F. ) ;
#9497=ADVANCED_FACE ( 'NONE', ( #3831 ), #2157, .T. ) ;
#9532=ORIENTED_EDGE ( 'NONE', *, *, #15128, .T. ) ;
#9534=ORIENTED_EDGE ( 'NONE', *, *, #13482, .T. ) ;
#9537=CARTESIAN_POINT ( 'NONE',  ( 20.49999999999998224, -21.99999999999999645, 11.00000000000000178 ) ) ;
#9543=LINE ( 'NONE', #14453, #12398 ) ;
#9554=VERTEX_POINT ( 'NONE', #5193 ) ;
#9558=ORIENTED_EDGE ( 'NONE', *, *, #1362, .T. ) ;
#9560=VERTEX_POINT ( 'NONE', #8237 ) ;
#9590=CARTESIAN_POINT ( 'NONE',  ( 11.00000000000000000, -23.83493649053891517, 4.999999999999999112 ) ) ;
#9596=ORIENTED_EDGE ( 'NONE', *, *, #4376, .T. ) ;
#9605=ORIENTED_EDGE ( 'NONE', *, *, #17075, .T. ) ;
#9633=EDGE_CURVE ( 'NONE', #3395, #4592, #16996, .T. ) ;
#9636=CARTESIAN_POINT ( 'NONE',  ( 11.00000000000000000, -23.70993649053891517, 5.466506350946108483 ) ) ;
#9656=VECTOR ( 'NONE', #12929, 1000.000000000000000 ) ;
#9659=AXIS2_PLACEMENT_3D ( 'NONE', #7999, #6540, #16055 ) ;
#9663=CIRCLE ( 'NONE', #15328, 2.500000000000000444 ) ;
#9664=EDGE_LOOP ( 'NONE', ( #2778, #16242, #12393, #15833 ) ) ;
#9668=CARTESIAN_POINT ( 'NONE',  ( -14.49999999999998579, -19.49999999999999645, 1.000000000000000000 ) ) ;
#9701=ADVANCED_FACE ( 'NONE', ( #2785, #10733 ), #9161, .F. ) ;
#9704=CYLINDRICAL_SURFACE ( 'NONE', #16885, 0.2500000000000002220 ) ;
#9715=AXIS2_PLACEMENT_3D ( 'NONE', #16887, #8848, #18570 ) ;
#9718=ORIENTED_EDGE ( 'NONE', *, *, #7952, .F. ) ;
#9720=ORIENTED_EDGE ( 'NONE', *, *, #15355, .F. ) ;
#9728=CARTESIAN_POINT ( 'NONE',  ( -13.49999999999998401, -21.99999999999999645, 14.18378559369222280 ) ) ;
#9773=VECTOR ( 'NONE', #10393, 1000.000000000000000 ) ;
#9781=LINE ( 'NONE', #8116, #7 ) ;
#9798=EDGE_CURVE ( 'NONE', #14709, #13635, #17509, .T. ) ;
#9810=VECTOR ( 'NONE', #5449, 1000.000000000000000 ) ;
#9823=ORIENTED_EDGE ( 'NONE', *, *, #1570, .F. ) ;
#9826=CARTESIAN_POINT ( 'NONE',  ( 0.000000000000000000, 0.000000000000000000, 4.000000000000000000 ) ) ;
#9846=DIRECTION ( 'NONE',  ( 1.000000000000000000, 0.000000000000000000, 0.000000000000000000 ) ) ;
#9851=VECTOR ( 'NONE', #13500, 1000.000000000000000 ) ;
#9859=LINE ( 'NONE', #1713, #2037 ) ;
#9872=PLANE ( 'NONE',  #1554 ) ;
#9885=VECTOR ( 'NONE', #6569, 1000.000000000000000 ) ;
#9898=EDGE_CURVE ( 'NONE', #7416, #3395, #17303, .T. ) ;
#9905=DIRECTION ( 'NONE',  ( -1.000000000000000000, 0.000000000000000000, 0.000000000000000000 ) ) ;
#9921=DIRECTION ( 'NONE',  ( -1.000000000000000000, -0.000000000000000000, 0.000000000000000000 ) ) ;
#9936=CARTESIAN_POINT ( 'NONE',  ( 20.49999999999998224, -21.99999999999999645, 9.999999999999998224 ) ) ;
#9963=ORIENTED_EDGE ( 'NONE', *, *, #154, .F. ) ;
#9972=EDGE_CURVE ( 'NONE', #20148, #19218, #14554, .T. ) ;
#9974=CARTESIAN_POINT ( 'NONE',  ( -14.49999999999998579, -25.49999999999999645, 4.000000000000000000 ) ) ;
#10001=VECTOR ( 'NONE', #14576, 1000.000000000000000 ) ;
#10052=CARTESIAN_POINT ( 'NONE',  ( 13.50000000000001243, -19.49999999999999645, 4.000000000000000000 ) ) ;
#10054=PLANE ( 'NONE',  #16798 ) ;
#10085=VECTOR ( 'NONE', #7856, 1000.000000000000000 ) ;
#10098=ORIENTED_EDGE ( 'NONE', *, *, #5955, .F. ) ;
#10107=ORIENTED_EDGE ( 'NONE', *, *, #528, .T. ) ;
#10109=CARTESIAN_POINT ( 'NONE',  ( -13.49999999999998401, -21.99999999999999645, 11.68378559369222280 ) ) ;
#10139=LINE ( 'NONE', #7110, #11794 ) ;
#10147=CARTESIAN_POINT ( 'NONE',  ( -2.499999999999998668, -19.50000000000000000, 1.000000000000000000 ) ) ;
#10162=EDGE_CURVE ( 'NONE', #17800, #3061, #5530, .T. ) ;
#10183=EDGE_CURVE ( 'NONE', #3797, #17356, #10652, .T. ) ;
#10187=CARTESIAN_POINT ( 'NONE',  ( -13.49999999999998401, -18.49999999999999645, 4.000000000000000000 ) ) ;
#10205=PLANE ( 'NONE',  #9715 ) ;
#10208=ORIENTED_EDGE ( 'NONE', *, *, #16334, .T. ) ;
#10224=EDGE_CURVE ( 'NONE', #3395, #15652, #7310, .T. ) ;
#10229=VERTEX_POINT ( 'NONE', #7520 ) ;
#10242=ORIENTED_EDGE ( 'NONE', *, *, #20429, .F. ) ;
#10247=CARTESIAN_POINT ( 'NONE',  ( -14.49999999999998579, -24.49999999999999289, 1.000000000000000000 ) ) ;
#10248=ORIENTED_EDGE ( 'NONE', *, *, #10789, .F. ) ;
#10254=DIRECTION ( 'NONE',  ( 0.000000000000000000, 1.000000000000000000, -0.000000000000000000 ) ) ;
#10283=DIRECTION ( 'NONE',  ( 1.000000000000000000, -0.000000000000000000, -0.000000000000000000 ) ) ;
#10305=VECTOR ( 'NONE', #3953, 1000.000000000000000 ) ;
#10322=LINE ( 'NONE', #16691, #12623 ) ;
#10337=VECTOR ( 'NONE', #14413, 1000.000000000000000 ) ;
#10339=LINE ( 'NONE', #13566, #7313 ) ;
#10340=ADVANCED_FACE ( 'NONE', ( #20596 ), #20393, .F. ) ;
#10343=DIRECTION ( 'NONE',  ( 0.000000000000000000, -1.000000000000000000, 0.000000000000000000 ) ) ;
#10344=DIRECTION ( 'NONE',  ( 8.673617379884047798E-17, -1.000000000000000000, 0.000000000000000000 ) ) ;
#10353=LINE ( 'NONE', #4391, #5070 ) ;
#10380=EDGE_CURVE ( 'NONE', #16077, #13777, #17541, .T. ) ;
#10387=LINE ( 'NONE', #12052, #1663 ) ;
#10388=VECTOR ( 'NONE', #11765, 1000.000000000000000 ) ;
#10393=DIRECTION ( 'NONE',  ( 0.000000000000000000, -1.000000000000000000, 0.000000000000000000 ) ) ;
#10394=CARTESIAN_POINT ( 'NONE',  ( -13.49999999999998401, -24.47992105705875332, 12.00000000000000000 ) ) ;
#10402=DIRECTION ( 'NONE',  ( -0.000000000000000000, 1.000000000000000000, -0.000000000000000000 ) ) ;
#10423=LINE ( 'NONE', #16793, #12911 ) ;
#10425=EDGE_CURVE ( 'NONE', #7379, #8351, #17442, .T. ) ;
#10448=EDGE_LOOP ( 'NONE', ( #2275, #19118, #1233, #267, #8819, #1096, #14007, #19221, #3414 ) ) ;
#10464=AXIS2_PLACEMENT_3D ( 'NONE', #20206, #12235, #18628 ) ;
#10490=DIRECTION ( 'NONE',  ( -1.000000000000000000, -0.000000000000000000, -0.000000000000000000 ) ) ;
#10495=AXIS2_PLACEMENT_3D ( 'NONE', #18997, #17731, #8215 ) ;
#10525=DIRECTION ( 'NONE',  ( 1.000000000000000000, 0.000000000000000000, -0.000000000000000000 ) ) ;
#10536=ORIENTED_EDGE ( 'NONE', *, *, #1538, .T. ) ;
#10541=ADVANCED_FACE ( 'NONE', ( #6871 ), #5195, .F. ) ;
#10546=EDGE_LOOP ( 'NONE', ( #9596, #17750, #16100, #3272 ) ) ;
#10552=EDGE_CURVE ( 'NONE', #6507, #5903, #13238, .T. ) ;
#10560=LINE ( 'NONE', #2495, #15428 ) ;
#10565=DIRECTION ( 'NONE',  ( 0.000000000000000000, 1.000000000000000000, 0.000000000000000000 ) ) ;
#10604=AXIS2_PLACEMENT_3D ( 'NONE', #3034, #17459, #11279 ) ;
#10609=ORIENTED_EDGE ( 'NONE', *, *, #19153, .F. ) ;
#10619=VERTEX_POINT ( 'NONE', #20448 ) ;
#10623=CARTESIAN_POINT ( 'NONE',  ( -14.49999999999998579, -21.99999999999999645, 9.999999999999998224 ) ) ;
#10640=EDGE_CURVE ( 'NONE', #11334, #12338, #15214, .T. ) ;
#10642=CARTESIAN_POINT ( 'NONE',  ( 11.00000000000000000, -20.16506350946107418, 5.250000000000000000 ) ) ;
#10646=VECTOR ( 'NONE', #17924, 1000.000000000000227 ) ;
#10650=VECTOR ( 'NONE', #17836, 1000.000000000000000 ) ;
#10652=LINE ( 'NONE', #13570, #9360 ) ;
#10656=DIRECTION ( 'NONE',  ( -1.000000000000000000, 0.000000000000000000, 0.000000000000000000 ) ) ;
#10668=AXIS2_PLACEMENT_3D ( 'NONE', #19039, #14000, #18933 ) ;
#10689=CIRCLE ( 'NONE', #12693, 1.000000000000002665 ) ;
#10690=LINE ( 'NONE', #18639, #17053 ) ;
#10706=LINE ( 'NONE', #17079, #18356 ) ;
#10708=PLANE ( 'NONE',  #464 ) ;
#10732=CARTESIAN_POINT ( 'NONE',  ( -7.499999999999999112, -25.49999999999999645, 4.000000000000000000 ) ) ;
#10733=FACE_OUTER_BOUND ( 'NONE', #12332, .T. ) ;
#10735=VECTOR ( 'NONE', #3068, 1000.000000000000000 ) ;
#10766=LINE ( 'NONE', #3501, #11353 ) ;
#10786=ORIENTED_EDGE ( 'NONE', *, *, #2352, .T. ) ;
#10789=EDGE_CURVE ( 'NONE', #12772, #14282, #2178, .T. ) ;
#10802=ORIENTED_EDGE ( 'NONE', *, *, #5914, .T. ) ;
#10808=ADVANCED_BREP_SHAPE_REPRESENTATION ( '', ( #17970, #18039 ), #15032 ) ;
#10822=AXIS2_PLACEMENT_3D ( 'NONE', #6081, #20210, #4406 ) ;
#10828=ORIENTED_EDGE ( 'NONE', *, *, #5658, .F. ) ;
#10834=ADVANCED_FACE ( 'NONE', ( #15871 ), #20506, .F. ) ;
#10887=ORIENTED_EDGE ( 'NONE', *, *, #5501, .T. ) ;
#10934=EDGE_LOOP ( 'NONE', ( #15685, #8744, #19735, #5185, #399, #1485 ) ) ;
#10939=DIRECTION ( 'NONE',  ( -8.673617379884045333E-17, 1.000000000000000000, 0.000000000000000000 ) ) ;
#10944=ADVANCED_FACE ( 'NONE', ( #5103 ), #1859, .T. ) ;
#10959=ADVANCED_FACE ( 'NONE', ( #14918 ), #9704, .T. ) ;
#10966=( GEOMETRIC_REPRESENTATION_CONTEXT ( 3 ) GLOBAL_UNCERTAINTY_ASSIGNED_CONTEXT ( ( #20125 ) ) GLOBAL_UNIT_ASSIGNED_CONTEXT ( ( #6364, #5101, #19136 ) ) REPRESENTATION_CONTEXT ( 'NONE', 'WORKASPACE' ) );
#10970=VECTOR ( 'NONE', #17434, 1000.000000000000000 ) ;
#10980=CYLINDRICAL_SURFACE ( 'NONE', #10604, 0.2500000000000002220 ) ;
#10997=VECTOR ( 'NONE', #8354, 1000.000000000000000 ) ;
#11027=DIRECTION ( 'NONE',  ( 0.000000000000000000, -0.9919684228235026158, 0.1264857625231113336 ) ) ;
#11038=EDGE_CURVE ( 'NONE', #3437, #16270, #11675, .T. ) ;
#11043=CARTESIAN_POINT ( 'NONE',  ( -14.49999999999998579, -18.49999999999999645, 4.000000000000000000 ) ) ;
#11063=VECTOR ( 'NONE', #1205, 1000.000000000000227 ) ;
#11088=ORIENTED_EDGE ( 'NONE', *, *, #12646, .F. ) ;
#11119=LINE ( 'NONE', #7971, #10735 ) ;
#11125=VERTEX_POINT ( 'NONE', #11579 ) ;
#11134=DIRECTION ( 'NONE',  ( 0.000000000000000000, 0.000000000000000000, 1.000000000000000000 ) ) ;
#11139=DIRECTION ( 'NONE',  ( 0.000000000000000000, 1.000000000000000000, -0.000000000000000000 ) ) ;
#11140=FACE_OUTER_BOUND ( 'NONE', #6433, .T. ) ;
#11143=PLANE ( 'NONE',  #20362 ) ;
#11179=ORIENTED_EDGE ( 'NONE', *, *, #12449, .T. ) ;
#11185=ORIENTED_EDGE ( 'NONE', *, *, #18314, .T. ) ;
#11188=ADVANCED_FACE ( 'NONE', ( #18275 ), #8862, .T. ) ;
#11217=CARTESIAN_POINT ( 'NONE',  ( -14.49999999999998579, -18.49999999999999645, 1.000000000000000000 ) ) ;
#11228=ORIENTED_EDGE ( 'NONE', *, *, #11944, .T. ) ;
#11231=CARTESIAN_POINT ( 'NONE',  ( -7.500000000000000000, -19.49999999999999645, 5.000000000000000000 ) ) ;
#11233=ORIENTED_EDGE ( 'NONE', *, *, #14713, .F. ) ;
#11236=DIRECTION ( 'NONE',  ( 8.673617379884045333E-17, -1.000000000000000000, 0.000000000000000000 ) ) ;
#11243=DIRECTION ( 'NONE',  ( 0.000000000000000000, 0.1264857625231113059, -0.9919684228235025047 ) ) ;
#11253=EDGE_LOOP ( 'NONE', ( #6467, #17376, #12658, #15006 ) ) ;
#11256=ORIENTED_EDGE ( 'NONE', *, *, #14213, .T. ) ;
#11258=ORIENTED_EDGE ( 'NONE', *, *, #19165, .T. ) ;
#11263=DIRECTION ( 'NONE',  ( 0.000000000000000000, -1.000000000000000000, 1.304178812473495102E-15 ) ) ;
#11277=CARTESIAN_POINT ( 'NONE',  ( -2.499999999999998224, -24.49999999999999289, 1.000000000000000000 ) ) ;
#11279=DIRECTION ( 'NONE',  ( 0.000000000000000000, 0.000000000000000000, 1.000000000000000000 ) ) ;
#11290=LINE ( 'NONE', #14316, #16688 ) ;
#11310=LINE ( 'NONE', #5237, #16048 ) ;
#11334=VERTEX_POINT ( 'NONE', #14178 ) ;
#11340=CARTESIAN_POINT ( 'NONE',  ( 7.499999999999999112, -25.49999999999999645, 4.000000000000000000 ) ) ;
#11343=VECTOR ( 'NONE', #896, 1000.000000000000000 ) ;
#11346=AXIS2_PLACEMENT_3D ( 'NONE', #16, #18755, #9224 ) ;
#11352=EDGE_CURVE ( 'NONE', #17295, #1310, #18910, .T. ) ;
#11353=VECTOR ( 'NONE', #14483, 1000.000000000000000 ) ;
#11363=( GEOMETRIC_REPRESENTATION_CONTEXT ( 3 ) GLOBAL_UNCERTAINTY_ASSIGNED_CONTEXT ( ( #12155 ) ) GLOBAL_UNIT_ASSIGNED_CONTEXT ( ( #6380, #12538, #20517 ) ) REPRESENTATION_CONTEXT ( 'NONE', 'WORKASPACE' ) );
#11384=VECTOR ( 'NONE', #19589, 1000.000000000000000 ) ;
#11394=CARTESIAN_POINT ( 'NONE',  ( -7.499999999999999112, -18.49999999999999645, 4.000000000000000000 ) ) ;
#11395=CARTESIAN_POINT ( 'NONE',  ( 14.50000000000001243, -18.49999999999999645, 1.000000000000000000 ) ) ;
#11396=AXIS2_PLACEMENT_3D ( 'NONE', #2116, #17908, #19592 ) ;
#11417=EDGE_CURVE ( 'NONE', #18461, #20067, #3109, .T. ) ;
#11453=CARTESIAN_POINT ( 'NONE',  ( -14.49999999999998579, -25.49999999999999645, 4.000000000000000000 ) ) ;
#11480=PRESENTATION_STYLE_ASSIGNMENT (( #6672 ) ) ;
#11496=ORIENTED_EDGE ( 'NONE', *, *, #858, .T. ) ;
#11503=DIRECTION ( 'NONE',  ( 0.000000000000000000, 0.000000000000000000, 1.000000000000000000 ) ) ;
#11512=VERTEX_POINT ( 'NONE', #14591 ) ;
#11513=VERTEX_POINT ( 'NONE', #3610 ) ;
#11515=CARTESIAN_POINT ( 'NONE',  ( -11.00000000000000000, -18.49999999999999645, 6.500000000000000888 ) ) ;
#11542=CARTESIAN_POINT ( 'NONE',  ( 7.499999999999999112, -24.49999999999999289, 5.000000000000000000 ) ) ;
#11545=LINE ( 'NONE', #16355, #1627 ) ;
#11574=CARTESIAN_POINT ( 'NONE',  ( 11.00000000000000000, -19.49999999999999645, 5.000000000000000000 ) ) ;
#11579=CARTESIAN_POINT ( 'NONE',  ( -13.49999999999998401, -19.49999999999999645, 4.000000000000000000 ) ) ;
#11585=ORIENTED_EDGE ( 'NONE', *, *, #809, .F. ) ;
#11594=CARTESIAN_POINT ( 'NONE',  ( -20.49999999999998224, -21.99999999999999645, 9.999999999999998224 ) ) ;
#11605=EDGE_CURVE ( 'NONE', #3437, #7178, #14699, .T. ) ;
#11612=VERTEX_POINT ( 'NONE', #8325 ) ;
#11641=EDGE_CURVE ( 'NONE', #1443, #6686, #15003, .T. ) ;
#11675=LINE ( 'NONE', #596, #9885 ) ;
#11684=EDGE_CURVE ( 'NONE', #2297, #16697, #13634, .T. ) ;
#11690=VECTOR ( 'NONE', #438, 1000.000000000000000 ) ;
#11696=CARTESIAN_POINT ( 'NONE',  ( -11.00000000000000000, -18.49999999999999645, 6.500000000000000888 ) ) ;
#11711=DIRECTION ( 'NONE',  ( 0.000000000000000000, 0.5000000000000037748, -0.8660254037844365982 ) ) ;
#11720=AXIS2_PLACEMENT_3D ( 'NONE', #17888, #16117, #13074 ) ;
#11745=EDGE_LOOP ( 'NONE', ( #7252, #3420, #296, #9532 ) ) ;
#11765=DIRECTION ( 'NONE',  ( -8.673617379884047798E-17, 1.000000000000000000, -0.000000000000000000 ) ) ;
#11794=VECTOR ( 'NONE', #10344, 1000.000000000000000 ) ;
#11820=( NAMED_UNIT ( * ) SI_UNIT ( $, .STERADIAN. ) SOLID_ANGLE_UNIT ( ) );
#11877=CARTESIAN_POINT ( 'NONE',  ( 14.49999999999998579, -21.99999999999999645, 12.00000000000000355 ) ) ;
#11919=( LENGTH_UNIT ( ) NAMED_UNIT ( * ) SI_UNIT ( .MILLI., .METRE. ) );
#11935=LINE ( 'NONE', #3994, #17381 ) ;
#11944=EDGE_CURVE ( 'NONE', #5816, #9416, #7581, .T. ) ;
#11953=DIRECTION ( 'NONE',  ( 0.000000000000000000, 1.000000000000000000, 0.000000000000000000 ) ) ;
#11954=DIRECTION ( 'NONE',  ( -0.000000000000000000, -0.000000000000000000, 1.000000000000000000 ) ) ;
#11956=CARTESIAN_POINT ( 'NONE',  ( 2.499999999999998668, -19.50000000000000000, 1.000000000000000000 ) ) ;
#11969=ORIENTED_EDGE ( 'NONE', *, *, #608, .T. ) ;
#11978=DIRECTION ( 'NONE',  ( 0.000000000000000000, 0.000000000000000000, 1.000000000000000000 ) ) ;
#11992=ORIENTED_EDGE ( 'NONE', *, *, #5534, .T. ) ;
#11996=CARTESIAN_POINT ( 'NONE',  ( -11.00000000000000000, -19.49999999999999645, 4.000000000000000000 ) ) ;
#11997=DIRECTION ( 'NONE',  ( -1.000000000000000000, -0.000000000000000000, -0.000000000000000000 ) ) ;
#12002=ORIENTED_EDGE ( 'NONE', *, *, #9260, .F. ) ;
#12019=CIRCLE ( 'NONE', #19710, 1.000000000000002665 ) ;
#12021=CARTESIAN_POINT ( 'NONE',  ( 11.00000000000000000, -18.49999999999999645, 6.500000000000000888 ) ) ;
#12022=VERTEX_POINT ( 'NONE', #7402 ) ;
#12052=CARTESIAN_POINT ( 'NONE',  ( 7.499999999999999112, -23.83493649053891517, 4.999999999999999112 ) ) ;
#12068=DIRECTION ( 'NONE',  ( 1.000000000000000000, 0.000000000000000000, -0.000000000000000000 ) ) ;
#12085=AXIS2_PLACEMENT_3D ( 'NONE', #13791, #18517, #7320 ) ;
#12096=EDGE_CURVE ( 'NONE', #13635, #18461, #9069, .T. ) ;
#12108=LINE ( 'NONE', #3947, #4988 ) ;
#12118=CARTESIAN_POINT ( 'NONE',  ( 14.49999999999998579, -19.52007894294123957, 12.00000000000000000 ) ) ;
#12127=VECTOR ( 'NONE', #20614, 1000.000000000000000 ) ;
#12131=ORIENTED_EDGE ( 'NONE', *, *, #7829, .T. ) ;
#12137=ORIENTED_EDGE ( 'NONE', *, *, #4541, .T. ) ;
#12141=CARTESIAN_POINT ( 'NONE',  ( 7.499999999999999112, -18.49999999999999645, 4.000000000000000000 ) ) ;
#12155=UNCERTAINTY_MEASURE_WITH_UNIT (LENGTH_MEASURE( 1.000000000000000082E-05 ), #6380, 'distance_accuracy_value', 'NONE');
#12156=ORIENTED_EDGE ( 'NONE', *, *, #17610, .F. ) ;
#12178=CARTESIAN_POINT ( 'NONE',  ( 11.00000000000000000, -24.49999999999999289, 5.000000000000000000 ) ) ;
#12181=PLANE ( 'NONE',  #4737 ) ;
#12188=CARTESIAN_POINT ( 'NONE',  ( -13.49999999999998401, -18.49999999999999645, 4.000000000000000000 ) ) ;
#12215=CARTESIAN_POINT ( 'NONE',  ( 7.499999999999999112, -25.49999999999999645, 4.000000000000000000 ) ) ;
#12235=DIRECTION ( 'NONE',  ( 1.000000000000000000, 0.000000000000000000, -0.000000000000000000 ) ) ;
#12242=DIRECTION ( 'NONE',  ( 0.000000000000000000, -1.000000000000000000, 0.000000000000000000 ) ) ;
#12255=ORIENTED_EDGE ( 'NONE', *, *, #7708, .T. ) ;
#12270=CYLINDRICAL_SURFACE ( 'NONE', #16723, 0.2500000000000002220 ) ;
#12301=AXIS2_PLACEMENT_3D ( 'NONE', #9265, #7702, #13761 ) ;
#12307=ORIENTED_EDGE ( 'NONE', *, *, #16479, .F. ) ;
#12314=LINE ( 'NONE', #18603, #10305 ) ;
#12332=EDGE_LOOP ( 'NONE', ( #1177, #11088, #6810, #13530, #217, #16049, #15752 ) ) ;
#12338=VERTEX_POINT ( 'NONE', #17165 ) ;
#12365=EDGE_CURVE ( 'NONE', #15652, #5903, #11935, .T. ) ;
#12381=CARTESIAN_POINT ( 'NONE',  ( 11.00000000000000000, -23.83493649053891517, 5.249999999999999112 ) ) ;
#12385=VERTEX_POINT ( 'NONE', #957 ) ;
#12389=PLANE ( 'NONE',  #18463 ) ;
#12393=ORIENTED_EDGE ( 'NONE', *, *, #7678, .T. ) ;
#12398=VECTOR ( 'NONE', #228, 1000.000000000000000 ) ;
#12423=DIRECTION ( 'NONE',  ( -0.000000000000000000, 1.000000000000000000, -0.000000000000000000 ) ) ;
#12426=LINE ( 'NONE', #4683, #2612 ) ;
#12436=CARTESIAN_POINT ( 'NONE',  ( -7.499999999999999112, -18.49999999999999645, 4.000000000000000000 ) ) ;
#12445=DIRECTION ( 'NONE',  ( -1.000000000000000000, -0.000000000000000000, -0.000000000000000000 ) ) ;
#12449=EDGE_CURVE ( 'NONE', #5966, #8747, #10690, .T. ) ;
#12456=CIRCLE ( 'NONE', #10464, 0.2500000000000002220 ) ;
#12478=AXIS2_PLACEMENT_3D ( 'NONE', #13276, #17896, #3775 ) ;
#12481=EDGE_LOOP ( 'NONE', ( #10609, #13802, #482, #7271 ) ) ;
#12497=CARTESIAN_POINT ( 'NONE',  ( 13.50000000000001243, -19.49999999999999645, 4.000000000000000000 ) ) ;
#12511=ORIENTED_EDGE ( 'NONE', *, *, #17922, .T. ) ;
#12522=CIRCLE ( 'NONE', #3187, 2.500000000000000444 ) ;
#12524=DIRECTION ( 'NONE',  ( 0.000000000000000000, -1.000000000000000000, 1.304178812473495102E-15 ) ) ;
#12538=( NAMED_UNIT ( * ) PLANE_ANGLE_UNIT ( ) SI_UNIT ( $, .RADIAN. ) );
#12560=PRODUCT_DEFINITION_CONTEXT ( 'detailed design', #12945, 'design' ) ;
#12563=FACE_OUTER_BOUND ( 'NONE', #12613, .T. ) ;
#12568=DIRECTION ( 'NONE',  ( 0.000000000000000000, 0.000000000000000000, -1.000000000000000000 ) ) ;
#12587=ORIENTED_EDGE ( 'NONE', *, *, #4935, .F. ) ;
#12609=DIRECTION ( 'NONE',  ( 1.000000000000000000, -0.000000000000000000, 0.000000000000000000 ) ) ;
#12612=DIRECTION ( 'NONE',  ( 0.000000000000000000, 1.000000000000000000, 0.000000000000000000 ) ) ;
#12613=EDGE_LOOP ( 'NONE', ( #4899, #19941, #1871, #11585, #10802, #15859 ) ) ;
#12623=VECTOR ( 'NONE', #13348, 1000.000000000000000 ) ;
#12638=VECTOR ( 'NONE', #13832, 1000.000000000000227 ) ;
#12644=CYLINDRICAL_SURFACE ( 'NONE', #10822, 0.2500000000000002220 ) ;
#12646=EDGE_CURVE ( 'NONE', #4544, #12022, #6280, .T. ) ;
#12649=AXIS2_PLACEMENT_3D ( 'NONE', #3286, #15936, #1616 ) ;
#12658=ORIENTED_EDGE ( 'NONE', *, *, #7111, .T. ) ;
#12663=CARTESIAN_POINT ( 'NONE',  ( -13.49999999999998401, -19.49999999999999645, 1.000000000000000000 ) ) ;
#12693=AXIS2_PLACEMENT_3D ( 'NONE', #2186, #5123, #11503 ) ;
#12695=CARTESIAN_POINT ( 'NONE',  ( 11.00000000000000000, -19.49999999999999645, 5.000000000000000000 ) ) ;
#12700=EDGE_CURVE ( 'NONE', #3061, #14333, #3456, .T. ) ;
#12728=CARTESIAN_POINT ( 'NONE',  ( -20.49999999999998224, -21.99999999999999645, 11.00000000000000178 ) ) ;
#12743=LINE ( 'NONE', #12436, #15288 ) ;
#12746=CARTESIAN_POINT ( 'NONE',  ( -3.499999999999998668, -19.50000000000000000, 1.000000000000000000 ) ) ;
#12754=LINE ( 'NONE', #11395, #467 ) ;
#12764=VECTOR ( 'NONE', #4655, 1000.000000000000000 ) ;
#12765=ADVANCED_FACE ( 'NONE', ( #14845 ), #1888, .T. ) ;
#12772=VERTEX_POINT ( 'NONE', #9936 ) ;
#12775=CARTESIAN_POINT ( 'NONE',  ( -7.500000000000000000, -20.16506350946107418, 5.000000000000000000 ) ) ;
#12797=VECTOR ( 'NONE', #15735, 1000.000000000000000 ) ;
#12798=EDGE_CURVE ( 'NONE', #19218, #16697, #2190, .T. ) ;
#12799=ORIENTED_EDGE ( 'NONE', *, *, #3105, .T. ) ;
#12805=DIRECTION ( 'NONE',  ( 0.000000000000000000, 0.000000000000000000, 1.000000000000000000 ) ) ;
#12823=DIRECTION ( 'NONE',  ( 1.000000000000000000, 0.000000000000000000, 0.000000000000000000 ) ) ;
#12824=EDGE_CURVE ( 'NONE', #20175, #483, #6403, .T. ) ;
#12825=ORIENTED_EDGE ( 'NONE', *, *, #1732, .T. ) ;
#12865=AXIS2_PLACEMENT_3D ( 'NONE', #14142, #20549, #20332 ) ;
#12874=VERTEX_POINT ( 'NONE', #20195 ) ;
#12895=CARTESIAN_POINT ( 'NONE',  ( -11.00000000000000000, -25.49999999999999645, 6.500000000000000000 ) ) ;
#12906=ADVANCED_FACE ( 'NONE', ( #15052 ), #2494, .F. ) ;
#12911=VECTOR ( 'NONE', #2673, 1000.000000000000000 ) ;
#12922=EDGE_LOOP ( 'NONE', ( #13177, #1790, #1025, #3538 ) ) ;
#12929=DIRECTION ( 'NONE',  ( 0.000000000000000000, 0.000000000000000000, -1.000000000000000000 ) ) ;
#12945=APPLICATION_CONTEXT ( 'automotive_design' ) ;
#12949=EDGE_CURVE ( 'NONE', #20223, #2296, #12743, .T. ) ;
#12970=ORIENTED_EDGE ( 'NONE', *, *, #19370, .T. ) ;
#12979=DIRECTION ( 'NONE',  ( -1.000000000000000000, 0.000000000000000000, 0.000000000000000000 ) ) ;
#12980=DIRECTION ( 'NONE',  ( 0.000000000000000000, 0.000000000000000000, 1.000000000000000000 ) ) ;
#13013=CARTESIAN_POINT ( 'NONE',  ( -2.499999999999998668, -19.50000000000000000, 1.000000000000000000 ) ) ;
#13017=CARTESIAN_POINT ( 'NONE',  ( 13.49999999999998401, -18.49999999999999645, 4.000000000000000000 ) ) ;
#13045=CARTESIAN_POINT ( 'NONE',  ( -7.499999999999999112, -18.49999999999999645, 6.500000000000000888 ) ) ;
#13047=EDGE_LOOP ( 'NONE', ( #4775, #2765, #4806, #4063 ) ) ;
#13056=VECTOR ( 'NONE', #7364, 1000.000000000000000 ) ;
#13074=DIRECTION ( 'NONE',  ( 0.000000000000000000, -0.000000000000000000, -1.000000000000000000 ) ) ;
#13091=LINE ( 'NONE', #13288, #5719 ) ;
#13096=VECTOR ( 'NONE', #20671, 1000.000000000000000 ) ;
#13120=LINE ( 'NONE', #16558, #8062 ) ;
#13122=CARTESIAN_POINT ( 'NONE',  ( -14.49999999999998579, -24.47992105705875332, 12.00000000000000000 ) ) ;
#13135=VERTEX_POINT ( 'NONE', #5308 ) ;
#13143=LINE ( 'NONE', #19541, #1303 ) ;
#13144=DIRECTION ( 'NONE',  ( -0.000000000000000000, 1.304178812473495102E-15, 1.000000000000000000 ) ) ;
#13151=VERTEX_POINT ( 'NONE', #14616 ) ;
#13172=ADVANCED_FACE ( 'NONE', ( #5737 ), #2270, .T. ) ;
#13177=ORIENTED_EDGE ( 'NONE', *, *, #7824, .F. ) ;
#13191=LINE ( 'NONE', #16630, #11384 ) ;
#13201=ORIENTED_EDGE ( 'NONE', *, *, #4151, .F. ) ;
#13207=CARTESIAN_POINT ( 'NONE',  ( 2.499999999999999112, -24.49999999999999289, 1.000000000000000000 ) ) ;
#13209=DIRECTION ( 'NONE',  ( 0.000000000000000000, 0.000000000000000000, 1.000000000000000000 ) ) ;
#13218=EDGE_CURVE ( 'NONE', #5898, #20661, #18394, .T. ) ;
#13230=CARTESIAN_POINT ( 'NONE',  ( 11.00000000000000000, -25.49999999999999645, 6.500000000000000000 ) ) ;
#13234=ORIENTED_EDGE ( 'NONE', *, *, #18702, .T. ) ;
#13237=LINE ( 'NONE', #13344, #6974 ) ;
#13238=LINE ( 'NONE', #11574, #9656 ) ;
#13259=VERTEX_POINT ( 'NONE', #11996 ) ;
#13272=PLANE ( 'NONE',  #1974 ) ;
#13276=CARTESIAN_POINT ( 'NONE',  ( -20.49999999999998224, -21.99999999999999645, 11.00000000000000178 ) ) ;
#13288=CARTESIAN_POINT ( 'NONE',  ( -14.49999999999998579, -19.49999999999999645, 4.000000000000000000 ) ) ;
#13302=EDGE_LOOP ( 'NONE', ( #268, #12131, #13789, #18136 ) ) ;
#13306=VECTOR ( 'NONE', #9183, 1000.000000000000000 ) ;
#13332=ORIENTED_EDGE ( 'NONE', *, *, #9414, .F. ) ;
#13344=CARTESIAN_POINT ( 'NONE',  ( -13.49999999999998401, -19.52007894294123957, 12.00000000000000000 ) ) ;
#13348=DIRECTION ( 'NONE',  ( 1.000000000000000000, -0.000000000000000000, 0.000000000000000000 ) ) ;
#13350=DIRECTION ( 'NONE',  ( 0.000000000000000000, -1.000000000000000000, 0.000000000000000000 ) ) ;
#13363=LINE ( 'NONE', #16504, #19164 ) ;
#13370=FACE_BOUND ( 'NONE', #15553, .T. ) ;
#13388=ORIENTED_EDGE ( 'NONE', *, *, #1360, .F. ) ;
#13416=CARTESIAN_POINT ( 'NONE',  ( -7.499999999999999112, -18.49999999999999645, 6.500000000000000888 ) ) ;
#13417=DIRECTION ( 'NONE',  ( 1.000000000000000000, 0.000000000000000000, 0.000000000000000000 ) ) ;
#13431=EDGE_CURVE ( 'NONE', #3175, #95, #1232, .T. ) ;
#13442=ADVANCED_FACE ( 'NONE', ( #4776 ), #6240, .T. ) ;
#13447=CARTESIAN_POINT ( 'NONE',  ( 11.00000000000000000, -18.49999999999999645, 4.000000000000000000 ) ) ;
#13462=DIRECTION ( 'NONE',  ( -0.000000000000000000, 1.000000000000000000, -0.000000000000000000 ) ) ;
#13465=ORIENTED_EDGE ( 'NONE', *, *, #13218, .F. ) ;
#13480=EDGE_CURVE ( 'NONE', #12338, #995, #17323, .T. ) ;
#13482=EDGE_CURVE ( 'NONE', #6507, #995, #7607, .T. ) ;
#13484=PLANE ( 'NONE',  #6748 ) ;
#13492=CARTESIAN_POINT ( 'NONE',  ( -3.499999999999998668, -19.50000000000000000, 4.000000000000000000 ) ) ;
#13493=SURFACE_STYLE_FILL_AREA ( #7130 ) ;
#13494=ORIENTED_EDGE ( 'NONE', *, *, #14213, .F. ) ;
#13498=LINE ( 'NONE', #2510, #4622 ) ;
#13500=DIRECTION ( 'NONE',  ( -1.000000000000000000, 0.000000000000000000, 0.000000000000000000 ) ) ;
#13515=DIRECTION ( 'NONE',  ( 0.000000000000000000, 1.000000000000000000, -1.304178812473495102E-15 ) ) ;
#13530=ORIENTED_EDGE ( 'NONE', *, *, #1596, .T. ) ;
#13540=ORIENTED_EDGE ( 'NONE', *, *, #1596, .F. ) ;
#13554=CARTESIAN_POINT ( 'NONE',  ( -14.49999999999998579, -19.49999999999999645, 4.000000000000000000 ) ) ;
#13566=CARTESIAN_POINT ( 'NONE',  ( 13.50000000000001243, -18.49999999999999645, 1.000000000000000000 ) ) ;
#13570=CARTESIAN_POINT ( 'NONE',  ( -13.49999999999998401, -24.49999999999999289, 4.000000000000000000 ) ) ;
#13608=EDGE_LOOP ( 'NONE', ( #13720, #6558, #13201, #16672 ) ) ;
#13619=CARTESIAN_POINT ( 'NONE',  ( 14.49999999999998579, -25.49999999999999645, 4.000000000000000000 ) ) ;
#13626=EDGE_LOOP ( 'NONE', ( #5343, #18572, #19787, #15620, #4074, #3815, #12970, #14077, #914, #4774, #9823, #18879, #1996, #7125 ) ) ;
#13634=LINE ( 'NONE', #13745, #10388 ) ;
#13635=VERTEX_POINT ( 'NONE', #3416 ) ;
#13637=ORIENTED_EDGE ( 'NONE', *, *, #12365, .F. ) ;
#13642=CARTESIAN_POINT ( 'NONE',  ( -14.49999999999998579, -19.52007894294123957, 12.00000000000000000 ) ) ;
#13645=CLOSED_SHELL ( 'NONE', ( #5426, #17692, #16399, #8273, #13442, #16767, #8210, #8095, #12765, #20591, #19263, #19734, #7368, #11188, #3900, #5528, #10541, #10834, #10959, #987, #16192, #16256, #9701, #13855, #14120, #2515, #14653, #14238, #10340, #34, #7984, #19280, #16021, #637, #13172, #17544, #8509, #7211, #4861, #10944, #12906, #19529, #8206, #926, #17194, #17455, #9497, #3933, #14158, #13837, #5318, #2456, #18507, #8612, #6928 ) ) ;
#13693=EDGE_CURVE ( 'NONE', #18235, #9195, #18055, .T. ) ;
#13720=ORIENTED_EDGE ( 'NONE', *, *, #1977, .T. ) ;
#13727=LINE ( 'NONE', #13619, #8717 ) ;
#13745=CARTESIAN_POINT ( 'NONE',  ( -2.499999999999998668, -19.50000000000000000, 4.000000000000000000 ) ) ;
#13747=ORIENTED_EDGE ( 'NONE', *, *, #18871, .F. ) ;
#13755=EDGE_CURVE ( 'NONE', #13151, #2226, #16376, .T. ) ;
#13757=DIRECTION ( 'NONE',  ( 0.000000000000000000, 0.000000000000000000, 1.000000000000000000 ) ) ;
#13761=DIRECTION ( 'NONE',  ( 0.000000000000000000, 0.000000000000000000, 1.000000000000000000 ) ) ;
#13774=LINE ( 'NONE', #4159, #18026 ) ;
#13777=VERTEX_POINT ( 'NONE', #14808 ) ;
#13789=ORIENTED_EDGE ( 'NONE', *, *, #9414, .T. ) ;
#13791=CARTESIAN_POINT ( 'NONE',  ( 20.49999999999998224, -21.99999999999999645, 11.00000000000000178 ) ) ;
#13797=VERTEX_POINT ( 'NONE', #15116 ) ;
#13802=ORIENTED_EDGE ( 'NONE', *, *, #19785, .T. ) ;
#13821=ORIENTED_EDGE ( 'NONE', *, *, #5657, .F. ) ;
#13832=DIRECTION ( 'NONE',  ( -0.000000000000000000, 0.1264857625231113059, -0.9919684228235025047 ) ) ;
#13837=ADVANCED_FACE ( 'NONE', ( #3825 ), #10205, .T. ) ;
#13847=ORIENTED_EDGE ( 'NONE', *, *, #17959, .T. ) ;
#13855=ADVANCED_FACE ( 'NONE', ( #16988, #15216 ), #12181, .F. ) ;
#13865=CIRCLE ( 'NONE', #3511, 0.2500000000000002220 ) ;
#13878=EDGE_LOOP ( 'NONE', ( #15556, #5626, #15955, #7131 ) ) ;
#13931=DIRECTION ( 'NONE',  ( -1.000000000000000000, -0.000000000000000000, -0.000000000000000000 ) ) ;
#13958=CARTESIAN_POINT ( 'NONE',  ( 11.00000000000000000, -19.49999999999999645, 5.000000000000000000 ) ) ;
#13964=CARTESIAN_POINT ( 'NONE',  ( -14.49999999999998579, -19.49999999999999645, 4.000000000000000000 ) ) ;
#13971=ORIENTED_EDGE ( 'NONE', *, *, #20088, .F. ) ;
#13974=EDGE_LOOP ( 'NONE', ( #3697, #840, #5938, #1159 ) ) ;
#13979=ORIENTED_EDGE ( 'NONE', *, *, #1308, .F. ) ;
#14000=DIRECTION ( 'NONE',  ( 1.000000000000000000, 0.000000000000000000, -0.000000000000000000 ) ) ;
#14007=ORIENTED_EDGE ( 'NONE', *, *, #10425, .F. ) ;
#14014=EDGE_CURVE ( 'NONE', #7416, #2967, #4342, .T. ) ;
#14016=CARTESIAN_POINT ( 'NONE',  ( -14.49999999999998579, -24.49999999999999289, 4.000000000000000000 ) ) ;
#14026=VERTEX_POINT ( 'NONE', #5908 ) ;
#14029=EDGE_LOOP ( 'NONE', ( #11185, #15649 ) ) ;
#14050=ORIENTED_EDGE ( 'NONE', *, *, #12096, .F. ) ;
#14077=ORIENTED_EDGE ( 'NONE', *, *, #1492, .F. ) ;
#14083=VECTOR ( 'NONE', #5951, 1000.000000000000000 ) ;
#14088=CARTESIAN_POINT ( 'NONE',  ( -11.00000000000000000, -19.49999999999999645, 4.000000000000000000 ) ) ;
#14089=DIRECTION ( 'NONE',  ( 0.000000000000000000, 0.000000000000000000, 1.000000000000000000 ) ) ;
#14099=EDGE_LOOP ( 'NONE', ( #5203, #18447, #7840, #6524 ) ) ;
#14120=ADVANCED_FACE ( 'NONE', ( #20250 ), #12389, .T. ) ;
#14135=ORIENTED_EDGE ( 'NONE', *, *, #9098, .F. ) ;
#14142=CARTESIAN_POINT ( 'NONE',  ( 20.49999999999998224, -21.99999999999999645, 11.00000000000000178 ) ) ;
#14143=DIRECTION ( 'NONE',  ( 0.000000000000000000, 0.000000000000000000, -1.000000000000000000 ) ) ;
#14158=ADVANCED_FACE ( 'NONE', ( #15622 ), #1307, .T. ) ;
#14178=CARTESIAN_POINT ( 'NONE',  ( 7.499999999999999112, -20.29006350946107418, 5.466506350946110260 ) ) ;
#14183=EDGE_CURVE ( 'NONE', #13635, #14476, #7129, .T. ) ;
#14184=ORIENTED_EDGE ( 'NONE', *, *, #19382, .F. ) ;
#14204=EDGE_LOOP ( 'NONE', ( #9963, #18150, #16375, #18374 ) ) ;
#14210=EDGE_CURVE ( 'NONE', #3840, #1310, #19677, .T. ) ;
#14213=EDGE_CURVE ( 'NONE', #15652, #14026, #16620, .T. ) ;
#14238=ADVANCED_FACE ( 'NONE', ( #15061 ), #3873, .F. ) ;
#14264=LINE ( 'NONE', #17514, #13096 ) ;
#14282=VERTEX_POINT ( 'NONE', #5233 ) ;
#14288=EDGE_CURVE ( 'NONE', #16270, #9560, #16735, .T. ) ;
#14296=DIRECTION ( 'NONE',  ( -1.000000000000000000, -0.000000000000000000, -0.000000000000000000 ) ) ;
#14316=CARTESIAN_POINT ( 'NONE',  ( 11.00000000000000000, -18.49999999999999645, 6.500000000000000888 ) ) ;
#14322=VECTOR ( 'NONE', #16614, 1000.000000000000000 ) ;
#14332=DIRECTION ( 'NONE',  ( 0.000000000000000000, -1.000000000000000000, 0.000000000000000000 ) ) ;
#14333=VERTEX_POINT ( 'NONE', #2102 ) ;
#14369=FACE_OUTER_BOUND ( 'NONE', #18523, .T. ) ;
#14390=CARTESIAN_POINT ( 'NONE',  ( 0.000000000000000000, 0.000000000000000000, 4.000000000000000000 ) ) ;
#14396=VECTOR ( 'NONE', #12242, 1000.000000000000000 ) ;
#14413=DIRECTION ( 'NONE',  ( 0.000000000000000000, 0.000000000000000000, 1.000000000000000000 ) ) ;
#14417=EDGE_LOOP ( 'NONE', ( #5304, #12825, #12255, #13234 ) ) ;
#14419=LINE ( 'NONE', #8055, #18153 ) ;
#14422=VECTOR ( 'NONE', #14296, 1000.000000000000000 ) ;
#14439=ORIENTED_EDGE ( 'NONE', *, *, #2109, .T. ) ;
#14445=ORIENTED_EDGE ( 'NONE', *, *, #13431, .T. ) ;
#14453=CARTESIAN_POINT ( 'NONE',  ( 11.00000000000000000, -25.49999999999999645, 4.000000000000000000 ) ) ;
#14462=CARTESIAN_POINT ( 'NONE',  ( -3.499999999999998668, -19.50000000000000000, 1.000000000000000000 ) ) ;
#14464=AXIS2_PLACEMENT_3D ( 'NONE', #9826, #16211, #14627 ) ;
#14472=ORIENTED_EDGE ( 'NONE', *, *, #1492, .T. ) ;
#14476=VERTEX_POINT ( 'NONE', #1158 ) ;
#14483=DIRECTION ( 'NONE',  ( -1.000000000000000000, 0.000000000000000000, 0.000000000000000000 ) ) ;
#14484=FACE_OUTER_BOUND ( 'NONE', #13047, .T. ) ;
#14497=ORIENTED_EDGE ( 'NONE', *, *, #5212, .T. ) ;
#14527=ORIENTED_EDGE ( 'NONE', *, *, #18401, .T. ) ;
#14533=DIRECTION ( 'NONE',  ( 1.000000000000000000, 0.000000000000000000, 0.000000000000000000 ) ) ;
#14548=ORIENTED_EDGE ( 'NONE', *, *, #15760, .F. ) ;
#14551=DIRECTION ( 'NONE',  ( 0.000000000000000000, 1.000000000000000000, 0.000000000000000000 ) ) ;
#14554=LINE ( 'NONE', #3759, #15357 ) ;
#14576=DIRECTION ( 'NONE',  ( -1.000000000000000000, 0.000000000000000000, 0.000000000000000000 ) ) ;
#14591=CARTESIAN_POINT ( 'NONE',  ( 13.49999999999998401, -25.49999999999999645, 4.000000000000000000 ) ) ;
#14616=CARTESIAN_POINT ( 'NONE',  ( -7.499999999999999112, -25.49999999999999645, 6.500000000000000888 ) ) ;
#14627=DIRECTION ( 'NONE',  ( 1.000000000000000000, 0.000000000000000000, 0.000000000000000000 ) ) ;
#14636=CARTESIAN_POINT ( 'NONE',  ( -11.00000000000000000, -23.83493649053891517, 4.999999999999999112 ) ) ;
#14648=CARTESIAN_POINT ( 'NONE',  ( 3.499999999999998668, -19.50000000000000000, 4.000000000000000000 ) ) ;
#14652=CARTESIAN_POINT ( 'NONE',  ( -11.00000000000000000, -24.49999999999999289, 5.000000000000000000 ) ) ;
#14653=ADVANCED_FACE ( 'NONE', ( #6265 ), #10980, .T. ) ;
#14671=ORIENTED_EDGE ( 'NONE', *, *, #16053, .F. ) ;
#14699=LINE ( 'NONE', #380, #16721 ) ;
#14709=VERTEX_POINT ( 'NONE', #12746 ) ;
#14713=EDGE_CURVE ( 'NONE', #11512, #8626, #7745, .T. ) ;
#14726=ORIENTED_EDGE ( 'NONE', *, *, #5440, .F. ) ;
#14755=CARTESIAN_POINT ( 'NONE',  ( 11.00000000000000000, -25.49999999999999645, 6.500000000000000000 ) ) ;
#14759=CARTESIAN_POINT ( 'NONE',  ( 14.50000000000001243, -18.49999999999999645, 4.000000000000000000 ) ) ;
#14760=CARTESIAN_POINT ( 'NONE',  ( -7.500000000000000000, -24.49999999999999289, 5.000000000000000000 ) ) ;
#14806=VERTEX_POINT ( 'NONE', #11594 ) ;
#14808=CARTESIAN_POINT ( 'NONE',  ( 11.00000000000000000, -24.49999999999999289, 4.000000000000000000 ) ) ;
#14814=LINE ( 'NONE', #2255, #15657 ) ;
#14815=DIRECTION ( 'NONE',  ( -0.000000000000000000, -0.000000000000000000, -1.000000000000000000 ) ) ;
#14820=DIRECTION ( 'NONE',  ( -1.000000000000000000, -0.000000000000000000, -0.000000000000000000 ) ) ;
#14845=FACE_OUTER_BOUND ( 'NONE', #16597, .T. ) ;
#14851=ORIENTED_EDGE ( 'NONE', *, *, #19357, .F. ) ;
#14855=ORIENTED_EDGE ( 'NONE', *, *, #7952, .T. ) ;
#14880=ORIENTED_EDGE ( 'NONE', *, *, #14713, .T. ) ;
#14882=DIRECTION ( 'NONE',  ( 1.000000000000000000, 0.000000000000000000, -0.000000000000000000 ) ) ;
#14883=DIRECTION ( 'NONE',  ( 0.000000000000000000, 0.000000000000000000, -1.000000000000000000 ) ) ;
#14894=AXIS2_PLACEMENT_3D ( 'NONE', #4753, #11139, #19513 ) ;
#14910=EDGE_CURVE ( 'NONE', #1310, #14026, #10339, .T. ) ;
#14918=FACE_OUTER_BOUND ( 'NONE', #13974, .T. ) ;
#14927=ORIENTED_EDGE ( 'NONE', *, *, #15655, .T. ) ;
#14936=DIRECTION ( 'NONE',  ( 0.000000000000000000, 0.000000000000000000, 1.000000000000000000 ) ) ;
#14945=LINE ( 'NONE', #321, #19774 ) ;
#15003=LINE ( 'NONE', #12178, #19416 ) ;
#15004=ORIENTED_EDGE ( 'NONE', *, *, #339, .T. ) ;
#15006=ORIENTED_EDGE ( 'NONE', *, *, #17922, .F. ) ;
#15007=DIRECTION ( 'NONE',  ( 0.000000000000000000, 0.000000000000000000, 1.000000000000000000 ) ) ;
#15011=LINE ( 'NONE', #17951, #973 ) ;
#15030=CARTESIAN_POINT ( 'NONE',  ( 3.499999999999998668, -19.50000000000000000, 4.000000000000000000 ) ) ;
#15032=( GEOMETRIC_REPRESENTATION_CONTEXT ( 3 ) GLOBAL_UNCERTAINTY_ASSIGNED_CONTEXT ( ( #15704 ) ) GLOBAL_UNIT_ASSIGNED_CONTEXT ( ( #11919, #1056, #11820 ) ) REPRESENTATION_CONTEXT ( 'NONE', 'WORKASPACE' ) );
#15052=FACE_OUTER_BOUND ( 'NONE', #6956, .T. ) ;
#15061=FACE_OUTER_BOUND ( 'NONE', #10546, .T. ) ;
#15064=CARTESIAN_POINT ( 'NONE',  ( 13.49999999999998401, -18.49999999999999645, 4.000000000000000000 ) ) ;
#15069=DIRECTION ( 'NONE',  ( 1.000000000000000000, 0.000000000000000000, 0.000000000000000000 ) ) ;
#15081=VERTEX_POINT ( 'NONE', #9281 ) ;
#15101=LINE ( 'NONE', #18040, #4974 ) ;
#15106=VECTOR ( 'NONE', #18112, 1000.000000000000114 ) ;
#15116=CARTESIAN_POINT ( 'NONE',  ( -3.499999999999997780, -24.49999999999999289, 1.000000000000000000 ) ) ;
#15118=ORIENTED_EDGE ( 'NONE', *, *, #55, .F. ) ;
#15128=EDGE_CURVE ( 'NONE', #13259, #12874, #6052, .T. ) ;
#15145=ORIENTED_EDGE ( 'NONE', *, *, #608, .F. ) ;
#15168=PRESENTATION_STYLE_ASSIGNMENT (( #8800 ) ) ;
#15190=ORIENTED_EDGE ( 'NONE', *, *, #6829, .F. ) ;
#15191=ORIENTED_EDGE ( 'NONE', *, *, #14910, .T. ) ;
#15195=CARTESIAN_POINT ( 'NONE',  ( -13.49999999999998401, -19.49999999999999645, 4.000000000000000000 ) ) ;
#15214=CIRCLE ( 'NONE', #17543, 0.2500000000000002220 ) ;
#15216=FACE_OUTER_BOUND ( 'NONE', #16345, .T. ) ;
#15224=DIRECTION ( 'NONE',  ( -0.000000000000000000, -0.000000000000000000, -1.000000000000000000 ) ) ;
#15225=AXIS2_PLACEMENT_3D ( 'NONE', #13554, #13350, #5829 ) ;
#15249=PLANE ( 'NONE',  #19504 ) ;
#15250=EDGE_CURVE ( 'NONE', #16077, #11512, #15011, .T. ) ;
#15288=VECTOR ( 'NONE', #9407, 1000.000000000000000 ) ;
#15328=AXIS2_PLACEMENT_3D ( 'NONE', #1162, #20521, #15480 ) ;
#15348=VERTEX_POINT ( 'NONE', #13642 ) ;
#15350=DIRECTION ( 'NONE',  ( 1.000000000000000000, -0.000000000000000000, 0.000000000000000000 ) ) ;
#15351=VECTOR ( 'NONE', #1803, 1000.000000000000000 ) ;
#15355=EDGE_CURVE ( 'NONE', #11612, #9195, #10423, .T. ) ;
#15357=VECTOR ( 'NONE', #7969, 1000.000000000000000 ) ;
#15376=VECTOR ( 'NONE', #3857, 1000.000000000000000 ) ;
#15399=EDGE_CURVE ( 'NONE', #1461, #12022, #9160, .T. ) ;
#15404=DIRECTION ( 'NONE',  ( 0.000000000000000000, 0.1264857625231113059, -0.9919684228235025047 ) ) ;
#15413=VERTEX_POINT ( 'NONE', #10732 ) ;
#15418=ORIENTED_EDGE ( 'NONE', *, *, #5623, .T. ) ;
#15428=VECTOR ( 'NONE', #7430, 1000.000000000000000 ) ;
#15450=DIRECTION ( 'NONE',  ( 1.000000000000000000, 0.000000000000000000, 0.000000000000000000 ) ) ;
#15456=CARTESIAN_POINT ( 'NONE',  ( -11.00000000000000000, -18.49999999999999645, 4.000000000000000000 ) ) ;
#15480=DIRECTION ( 'NONE',  ( 0.000000000000000000, 0.000000000000000000, -1.000000000000000000 ) ) ;
#15493=ORIENTED_EDGE ( 'NONE', *, *, #809, .T. ) ;
#15505=CARTESIAN_POINT ( 'NONE',  ( -14.49999999999998579, -24.49999999999999289, 4.000000000000000000 ) ) ;
#15506=DIRECTION ( 'NONE',  ( 0.000000000000000000, 0.000000000000000000, -1.000000000000000000 ) ) ;
#15533=DIRECTION ( 'NONE',  ( 0.000000000000000000, -1.000000000000000000, 0.000000000000000000 ) ) ;
#15539=LINE ( 'NONE', #5826, #16383 ) ;
#15551=ORIENTED_EDGE ( 'NONE', *, *, #16334, .F. ) ;
#15553=EDGE_LOOP ( 'NONE', ( #12307, #8736, #15551, #4477 ) ) ;
#15556=ORIENTED_EDGE ( 'NONE', *, *, #20468, .F. ) ;
#15562=DIRECTION ( 'NONE',  ( 1.000000000000000000, -0.000000000000000000, -0.000000000000000000 ) ) ;
#15620=ORIENTED_EDGE ( 'NONE', *, *, #7708, .F. ) ;
#15622=FACE_OUTER_BOUND ( 'NONE', #6378, .T. ) ;
#15626=DIRECTION ( 'NONE',  ( 0.000000000000000000, 0.000000000000000000, 1.000000000000000000 ) ) ;
#15649=ORIENTED_EDGE ( 'NONE', *, *, #12824, .T. ) ;
#15650=AXIS2_PLACEMENT_3D ( 'NONE', #14390, #6460, #12823 ) ;
#15652=VERTEX_POINT ( 'NONE', #12497 ) ;
#15655=EDGE_CURVE ( 'NONE', #8351, #2127, #12522, .T. ) ;
#15657=VECTOR ( 'NONE', #390, 1000.000000000000000 ) ;
#15661=VECTOR ( 'NONE', #15744, 1000.000000000000000 ) ;
#15683=LINE ( 'NONE', #1669, #17807 ) ;
#15685=ORIENTED_EDGE ( 'NONE', *, *, #7678, .F. ) ;
#15704=UNCERTAINTY_MEASURE_WITH_UNIT (LENGTH_MEASURE( 1.000000000000000082E-05 ), #11919, 'distance_accuracy_value', 'NONE');
#15706=PLANE ( 'NONE',  #16457 ) ;
#15719=ORIENTED_EDGE ( 'NONE', *, *, #11605, .T. ) ;
#15735=DIRECTION ( 'NONE',  ( 0.000000000000000000, -0.8660254037844363761, 0.5000000000000041078 ) ) ;
#15744=DIRECTION ( 'NONE',  ( -1.000000000000000000, 0.000000000000000000, 0.000000000000000000 ) ) ;
#15752=ORIENTED_EDGE ( 'NONE', *, *, #16816, .T. ) ;
#15760=EDGE_CURVE ( 'NONE', #9416, #9078, #950, .T. ) ;
#15761=EDGE_CURVE ( 'NONE', #8747, #18643, #13865, .T. ) ;
#15790=DIRECTION ( 'NONE',  ( -0.000000000000000000, -1.000000000000000000, 0.000000000000000000 ) ) ;
#15801=CARTESIAN_POINT ( 'NONE',  ( -20.49999999999998224, -21.99999999999999645, 12.00000000000000355 ) ) ;
#15833=ORIENTED_EDGE ( 'NONE', *, *, #3105, .F. ) ;
#15859=ORIENTED_EDGE ( 'NONE', *, *, #15862, .T. ) ;
#15862=EDGE_CURVE ( 'NONE', #2296, #17379, #8493, .T. ) ;
#15871=FACE_OUTER_BOUND ( 'NONE', #20140, .T. ) ;
#15879=LINE ( 'NONE', #3439, #10337 ) ;
#15936=DIRECTION ( 'NONE',  ( -1.000000000000000000, -0.000000000000000000, 0.000000000000000000 ) ) ;
#15954=EDGE_LOOP ( 'NONE', ( #7790, #5486, #13494, #7297, #4953, #9534, #7891, #5603 ) ) ;
#15955=ORIENTED_EDGE ( 'NONE', *, *, #2861, .T. ) ;
#15960=VECTOR ( 'NONE', #5715, 1000.000000000000000 ) ;
#15986=VERTEX_POINT ( 'NONE', #18738 ) ;
#16021=ADVANCED_FACE ( 'NONE', ( #20420 ), #12644, .T. ) ;
#16047=ORIENTED_EDGE ( 'NONE', *, *, #20231, .T. ) ;
#16048=VECTOR ( 'NONE', #14551, 1000.000000000000000 ) ;
#16049=ORIENTED_EDGE ( 'NONE', *, *, #18891, .T. ) ;
#16052=DIRECTION ( 'NONE',  ( -1.000000000000000000, 0.000000000000000000, 0.000000000000000000 ) ) ;
#16053=EDGE_CURVE ( 'NONE', #19576, #2967, #12754, .T. ) ;
#16055=DIRECTION ( 'NONE',  ( 1.734723475976809067E-16, -1.000000000000000000, 0.000000000000000000 ) ) ;
#16058=CARTESIAN_POINT ( 'NONE',  ( 11.00000000000000000, -18.49999999999999645, 6.500000000000000888 ) ) ;
#16074=ORIENTED_EDGE ( 'NONE', *, *, #1538, .F. ) ;
#16077=VERTEX_POINT ( 'NONE', #4705 ) ;
#16097=ORIENTED_EDGE ( 'NONE', *, *, #14288, .F. ) ;
#16100=ORIENTED_EDGE ( 'NONE', *, *, #3482, .F. ) ;
#16112=DIRECTION ( 'NONE',  ( 1.000000000000000000, -0.000000000000000000, 0.000000000000000000 ) ) ;
#16117=DIRECTION ( 'NONE',  ( 0.000000000000000000, -1.000000000000000000, 0.000000000000000000 ) ) ;
#16130=LINE ( 'NONE', #1899, #4023 ) ;
#16151=ORIENTED_EDGE ( 'NONE', *, *, #5100, .F. ) ;
#16168=DIRECTION ( 'NONE',  ( -1.000000000000000000, -0.000000000000000000, -0.000000000000000000 ) ) ;
#16192=ADVANCED_FACE ( 'NONE', ( #19256 ), #3448, .T. ) ;
#16211=DIRECTION ( 'NONE',  ( -0.000000000000000000, 0.000000000000000000, 1.000000000000000000 ) ) ;
#16214=DIRECTION ( 'NONE',  ( -1.000000000000000000, -0.000000000000000000, -0.000000000000000000 ) ) ;
#16225=ORIENTED_EDGE ( 'NONE', *, *, #8902, .F. ) ;
#16229=DIRECTION ( 'NONE',  ( 0.000000000000000000, 0.000000000000000000, 1.000000000000000000 ) ) ;
#16233=CARTESIAN_POINT ( 'NONE',  ( 13.49999999999998401, -25.49999999999999645, 4.000000000000000000 ) ) ;
#16242=ORIENTED_EDGE ( 'NONE', *, *, #1806, .T. ) ;
#16256=ADVANCED_FACE ( 'NONE', ( #13370, #19773, #19564, #5634 ), #15249, .F. ) ;
#16270=VERTEX_POINT ( 'NONE', #11696 ) ;
#16298=CARTESIAN_POINT ( 'NONE',  ( -14.49999999999998579, -18.49999999999999645, 4.000000000000000000 ) ) ;
#16300=ORIENTED_EDGE ( 'NONE', *, *, #2362, .F. ) ;
#16334=EDGE_CURVE ( 'NONE', #20148, #6837, #10139, .T. ) ;
#16345=EDGE_LOOP ( 'NONE', ( #19432, #5258, #13979, #18931, #2985, #14472 ) ) ;
#16355=CARTESIAN_POINT ( 'NONE',  ( -7.500000000000000000, -23.83493649053891517, 4.999999999999999112 ) ) ;
#16358=FACE_OUTER_BOUND ( 'NONE', #18159, .T. ) ;
#16375=ORIENTED_EDGE ( 'NONE', *, *, #12700, .T. ) ;
#16376=LINE ( 'NONE', #13230, #18771 ) ;
#16382=CARTESIAN_POINT ( 'NONE',  ( -13.49999999999998401, -18.49999999999999645, 4.000000000000000000 ) ) ;
#16383=VECTOR ( 'NONE', #2995, 1000.000000000000000 ) ;
#16397=VECTOR ( 'NONE', #17574, 1000.000000000000000 ) ;
#16398=ORIENTED_EDGE ( 'NONE', *, *, #10224, .F. ) ;
#16399=ADVANCED_FACE ( 'NONE', ( #5531 ), #923, .T. ) ;
#16410=CARTESIAN_POINT ( 'NONE',  ( -13.49999999999998401, -21.99999999999999645, 11.68378559369222280 ) ) ;
#16414=CARTESIAN_POINT ( 'NONE',  ( 20.49999999999998224, -21.99999999999999645, 11.00000000000000178 ) ) ;
#16454=EDGE_CURVE ( 'NONE', #8626, #1180, #9186, .T. ) ;
#16457=AXIS2_PLACEMENT_3D ( 'NONE', #4616, #1390, #7772 ) ;
#16462=CARTESIAN_POINT ( 'NONE',  ( -13.49999999999998401, -24.49999999999999289, 1.000000000000000000 ) ) ;
#16479=EDGE_CURVE ( 'NONE', #7462, #19218, #20081, .T. ) ;
#16485=DIRECTION ( 'NONE',  ( -1.000000000000000000, 0.000000000000000000, 0.000000000000000000 ) ) ;
#16486=DIRECTION ( 'NONE',  ( -1.000000000000000000, 0.000000000000000000, 0.000000000000000000 ) ) ;
#16504=CARTESIAN_POINT ( 'NONE',  ( -7.499999999999999112, -18.49999999999999645, 4.000000000000000000 ) ) ;
#16521=CARTESIAN_POINT ( 'NONE',  ( -7.499999999999999112, -25.49999999999999645, 6.500000000000000888 ) ) ;
#16526=ORIENTED_EDGE ( 'NONE', *, *, #18891, .F. ) ;
#16538=PLANE ( 'NONE',  #18757 ) ;
#16557=DIRECTION ( 'NONE',  ( 0.000000000000000000, 0.9919684228235026158, 0.1264857625231113336 ) ) ;
#16558=CARTESIAN_POINT ( 'NONE',  ( 11.00000000000000000, -23.70993649053891517, 5.466506350946108483 ) ) ;
#16567=EDGE_LOOP ( 'NONE', ( #14927, #7656, #13540, #17553 ) ) ;
#16594=VERTEX_POINT ( 'NONE', #12118 ) ;
#16597=EDGE_LOOP ( 'NONE', ( #15118, #19061, #19631, #7080, #11496, #5414, #13847, #220 ) ) ;
#16604=FACE_OUTER_BOUND ( 'NONE', #4856, .T. ) ;
#16611=DIRECTION ( 'NONE',  ( 0.000000000000000000, 0.9919684228235026158, -0.1264857625231113336 ) ) ;
#16614=DIRECTION ( 'NONE',  ( 1.000000000000000000, -0.000000000000000000, 0.000000000000000000 ) ) ;
#16620=LINE ( 'NONE', #10052, #9810 ) ;
#16628=DIRECTION ( 'NONE',  ( -1.000000000000000000, 0.000000000000000000, 0.000000000000000000 ) ) ;
#16630=CARTESIAN_POINT ( 'NONE',  ( -13.49999999999998401, -18.49999999999999645, 4.000000000000000000 ) ) ;
#16649=CARTESIAN_POINT ( 'NONE',  ( -13.49999999999998401, -24.47992105705875332, 12.00000000000000000 ) ) ;
#16654=DIRECTION ( 'NONE',  ( 0.000000000000000000, 0.000000000000000000, -1.000000000000000000 ) ) ;
#16672=ORIENTED_EDGE ( 'NONE', *, *, #55, .T. ) ;
#16683=DIRECTION ( 'NONE',  ( 1.000000000000000000, 0.000000000000000000, -0.000000000000000000 ) ) ;
#16685=DIRECTION ( 'NONE',  ( 0.000000000000000000, 0.000000000000000000, 1.000000000000000000 ) ) ;
#16688=VECTOR ( 'NONE', #1376, 1000.000000000000000 ) ;
#16691=CARTESIAN_POINT ( 'NONE',  ( -14.49999999999998579, -24.49999999999999289, 4.000000000000000000 ) ) ;
#16697=VERTEX_POINT ( 'NONE', #19234 ) ;
#16714=DIRECTION ( 'NONE',  ( -1.000000000000000000, 0.000000000000000000, 0.000000000000000000 ) ) ;
#16721=VECTOR ( 'NONE', #1941, 1000.000000000000114 ) ;
#16723=AXIS2_PLACEMENT_3D ( 'NONE', #12381, #18664, #7677 ) ;
#16725=ORIENTED_EDGE ( 'NONE', *, *, #795, .T. ) ;
#16731=CARTESIAN_POINT ( 'NONE',  ( -14.49999999999998579, -25.49999999999999645, 4.000000000000000000 ) ) ;
#16733=EDGE_LOOP ( 'NONE', ( #17579, #11969, #11179, #768, #3336, #7176 ) ) ;
#16735=LINE ( 'NONE', #11515, #15106 ) ;
#16767=ADVANCED_FACE ( 'NONE', ( #3932 ), #17955, .T. ) ;
#16778=VECTOR ( 'NONE', #3668, 1000.000000000000000 ) ;
#16793=CARTESIAN_POINT ( 'NONE',  ( 7.499999999999999112, -25.49999999999999645, 6.500000000000000888 ) ) ;
#16798=AXIS2_PLACEMENT_3D ( 'NONE', #2301, #10254, #5141 ) ;
#16810=DIRECTION ( 'NONE',  ( 0.000000000000000000, 0.000000000000000000, -1.000000000000000000 ) ) ;
#16816=EDGE_CURVE ( 'NONE', #9078, #1461, #5722, .T. ) ;
#16834=DIRECTION ( 'NONE',  ( 1.000000000000000000, 0.000000000000000000, 0.000000000000000000 ) ) ;
#16885=AXIS2_PLACEMENT_3D ( 'NONE', #3532, #14820, #17762 ) ;
#16887=CARTESIAN_POINT ( 'NONE',  ( -20.49999999999998224, -21.99999999999999645, 11.00000000000000178 ) ) ;
#16920=CARTESIAN_POINT ( 'NONE',  ( 13.49999999999998401, -18.49999999999999645, 4.000000000000000000 ) ) ;
#16933=DIRECTION ( 'NONE',  ( 0.000000000000000000, -0.000000000000000000, 1.000000000000000000 ) ) ;
#16988=FACE_BOUND ( 'NONE', #14029, .T. ) ;
#16989=AXIS2_PLACEMENT_3D ( 'NONE', #17084, #12068, #4220 ) ;
#16996=LINE ( 'NONE', #694, #11343 ) ;
#17053=VECTOR ( 'NONE', #4305, 1000.000000000000114 ) ;
#17073=PLANE ( 'NONE',  #3769 ) ;
#17075=EDGE_CURVE ( 'NONE', #1180, #16594, #5521, .T. ) ;
#17079=CARTESIAN_POINT ( 'NONE',  ( 14.49999999999998579, -18.49999999999999645, 4.000000000000000000 ) ) ;
#17084=CARTESIAN_POINT ( 'NONE',  ( 11.00000000000000000, -23.83493649053891517, 5.249999999999999112 ) ) ;
#17098=DIRECTION ( 'NONE',  ( -0.000000000000000000, -0.000000000000000000, -1.000000000000000000 ) ) ;
#17101=VECTOR ( 'NONE', #3027, 1000.000000000000000 ) ;
#17103=ORIENTED_EDGE ( 'NONE', *, *, #19165, .F. ) ;
#17105=DIRECTION ( 'NONE',  ( -0.000000000000000000, 0.000000000000000000, -1.000000000000000000 ) ) ;
#17123=CARTESIAN_POINT ( 'NONE',  ( 11.00000000000000000, -19.49999999999999645, 5.000000000000000000 ) ) ;
#17136=DIRECTION ( 'NONE',  ( 0.000000000000000000, 0.5000000000000037748, -0.8660254037844365982 ) ) ;
#17139=EDGE_LOOP ( 'NONE', ( #4488, #16074, #14671, #20076 ) ) ;
#17152=ORIENTED_EDGE ( 'NONE', *, *, #2203, .F. ) ;
#17165=CARTESIAN_POINT ( 'NONE',  ( 7.499999999999999112, -20.16506350946107418, 5.000000000000000000 ) ) ;
#17175=ORIENTED_EDGE ( 'NONE', *, *, #19264, .T. ) ;
#17194=ADVANCED_FACE ( 'NONE', ( #4654 ), #9367, .T. ) ;
#17196=CARTESIAN_POINT ( 'NONE',  ( -13.49999999999998401, -18.49999999999999645, 4.000000000000000000 ) ) ;
#17202=PLANE ( 'NONE',  #4462 ) ;
#17213=AXIS2_PLACEMENT_3D ( 'NONE', #1654, #17136, #2815 ) ;
#17264=ORIENTED_EDGE ( 'NONE', *, *, #10380, .T. ) ;
#17267=CARTESIAN_POINT ( 'NONE',  ( -20.49999999999998224, -21.99999999999999645, 12.00000000000000355 ) ) ;
#17282=EDGE_CURVE ( 'NONE', #6562, #3751, #5372, .T. ) ;
#17295=VERTEX_POINT ( 'NONE', #5073 ) ;
#17300=COLOUR_RGB ( '', 0.40784314, 0.44705882, 0.49803922) ;
#17303=LINE ( 'NONE', #11043, #3672 ) ;
#17323=LINE ( 'NONE', #1639, #1950 ) ;
#17326=AXIS2_PLACEMENT_3D ( 'NONE', #18379, #4142, #10525 ) ;
#17336=CARTESIAN_POINT ( 'NONE',  ( -2.499999999999998668, -19.50000000000000000, 1.000000000000000000 ) ) ;
#17356=VERTEX_POINT ( 'NONE', #16462 ) ;
#17376=ORIENTED_EDGE ( 'NONE', *, *, #5100, .T. ) ;
#17379=VERTEX_POINT ( 'NONE', #2136 ) ;
#17381=VECTOR ( 'NONE', #859, 1000.000000000000000 ) ;
#17410=FACE_OUTER_BOUND ( 'NONE', #8018, .T. ) ;
#17418=PLANE ( 'NONE',  #9659 ) ;
#17434=DIRECTION ( 'NONE',  ( -1.000000000000000000, -0.000000000000000000, -0.000000000000000000 ) ) ;
#17442=LINE ( 'NONE', #3121, #3021 ) ;
#17455=ADVANCED_FACE ( 'NONE', ( #16358 ), #3809, .T. ) ;
#17459=DIRECTION ( 'NONE',  ( -1.000000000000000000, -0.000000000000000000, -0.000000000000000000 ) ) ;
#17464=VERTEX_POINT ( 'NONE', #2648 ) ;
#17489=LINE ( 'NONE', #11217, #15351 ) ;
#17508=PLANE ( 'NONE',  #12649 ) ;
#17509=LINE ( 'NONE', #4457, #20710 ) ;
#17514=CARTESIAN_POINT ( 'NONE',  ( 11.00000000000000000, -23.83493649053891517, 4.999999999999999112 ) ) ;
#17517=CARTESIAN_POINT ( 'NONE',  ( 11.00000000000000000, -20.16506350946107418, 5.000000000000000000 ) ) ;
#17541=LINE ( 'NONE', #7826, #20691 ) ;
#17543=AXIS2_PLACEMENT_3D ( 'NONE', #18766, #18968, #15506 ) ;
#17544=ADVANCED_FACE ( 'NONE', ( #7366 ), #10708, .F. ) ;
#17550=EDGE_CURVE ( 'NONE', #18643, #6507, #4218, .T. ) ;
#17551=LINE ( 'NONE', #6164, #14422 ) ;
#17553=ORIENTED_EDGE ( 'NONE', *, *, #6694, .F. ) ;
#17556=FACE_OUTER_BOUND ( 'NONE', #741, .T. ) ;
#17562=CARTESIAN_POINT ( 'NONE',  ( -14.49999999999998579, -24.49999999999999289, 4.000000000000000000 ) ) ;
#17574=DIRECTION ( 'NONE',  ( -0.000000000000000000, -0.000000000000000000, -1.000000000000000000 ) ) ;
#17579=ORIENTED_EDGE ( 'NONE', *, *, #3053, .T. ) ;
#17593=DIRECTION ( 'NONE',  ( -1.000000000000000000, 0.000000000000000000, 0.000000000000000000 ) ) ;
#17599=ORIENTED_EDGE ( 'NONE', *, *, #14288, .T. ) ;
#17601=DIRECTION ( 'NONE',  ( 1.000000000000000000, 0.000000000000000000, 0.000000000000000000 ) ) ;
#17610=EDGE_CURVE ( 'NONE', #20090, #6562, #18456, .T. ) ;
#17613=FACE_OUTER_BOUND ( 'NONE', #7428, .T. ) ;
#17615=LINE ( 'NONE', #9668, #17990 ) ;
#17616=DIRECTION ( 'NONE',  ( 0.000000000000000000, 0.000000000000000000, 1.000000000000000000 ) ) ;
#17651=ORIENTED_EDGE ( 'NONE', *, *, #5955, .T. ) ;
#17678=VECTOR ( 'NONE', #20361, 1000.000000000000000 ) ;
#17691=ORIENTED_EDGE ( 'NONE', *, *, #17550, .F. ) ;
#17692=ADVANCED_FACE ( 'NONE', ( #6520 ), #2960, .T. ) ;
#17693=ORIENTED_EDGE ( 'NONE', *, *, #16816, .F. ) ;
#17731=DIRECTION ( 'NONE',  ( -1.000000000000000000, -0.000000000000000000, -0.000000000000000000 ) ) ;
#17750=ORIENTED_EDGE ( 'NONE', *, *, #8015, .T. ) ;
#17762=DIRECTION ( 'NONE',  ( 0.000000000000000000, 0.000000000000000000, 1.000000000000000000 ) ) ;
#17765=ORIENTED_EDGE ( 'NONE', *, *, #18314, .F. ) ;
#17769=ORIENTED_EDGE ( 'NONE', *, *, #11352, .F. ) ;
#17777=ORIENTED_EDGE ( 'NONE', *, *, #18619, .T. ) ;
#17783=DIRECTION ( 'NONE',  ( 0.000000000000000000, 0.000000000000000000, -1.000000000000000000 ) ) ;
#17789=DIRECTION ( 'NONE',  ( -0.000000000000000000, 1.000000000000000000, -1.304178812473495102E-15 ) ) ;
#17800=VERTEX_POINT ( 'NONE', #20502 ) ;
#17807=VECTOR ( 'NONE', #12445, 1000.000000000000000 ) ;
#17829=CARTESIAN_POINT ( 'NONE',  ( -11.00000000000000000, -20.16506350946107418, 5.250000000000000000 ) ) ;
#17836=DIRECTION ( 'NONE',  ( 1.000000000000000000, 0.000000000000000000, 0.000000000000000000 ) ) ;
#17862=DIRECTION ( 'NONE',  ( 1.000000000000000000, 0.000000000000000000, -0.000000000000000000 ) ) ;
#17888=CARTESIAN_POINT ( 'NONE',  ( -14.49999999999998579, -19.49999999999999645, 4.000000000000000000 ) ) ;
#17896=DIRECTION ( 'NONE',  ( 1.000000000000000000, -0.000000000000000000, -0.000000000000000000 ) ) ;
#17908=DIRECTION ( 'NONE',  ( -1.000000000000000000, 0.000000000000000000, 0.000000000000000000 ) ) ;
#17922=EDGE_CURVE ( 'NONE', #14806, #814, #12426, .T. ) ;
#17924=DIRECTION ( 'NONE',  ( 0.000000000000000000, 0.1264857625231113059, 0.9919684228235025047 ) ) ;
#17935=ORIENTED_EDGE ( 'NONE', *, *, #15760, .T. ) ;
#17951=CARTESIAN_POINT ( 'NONE',  ( -14.49999999999998579, -25.49999999999999645, 4.000000000000000000 ) ) ;
#17955=PLANE ( 'NONE',  #3285 ) ;
#17959=EDGE_CURVE ( 'NONE', #13259, #11125, #3530, .T. ) ;
#17970=MANIFOLD_SOLID_BREP ( 'Mirror1', #13645 ) ;
#17990=VECTOR ( 'NONE', #16052, 1000.000000000000000 ) ;
#18026=VECTOR ( 'NONE', #11134, 1000.000000000000000 ) ;
#18031=FACE_OUTER_BOUND ( 'NONE', #7149, .T. ) ;
#18039=AXIS2_PLACEMENT_3D ( 'NONE', #1793, #16229, #8180 ) ;
#18040=CARTESIAN_POINT ( 'NONE',  ( -11.00000000000000000, -24.49999999999999289, 4.000000000000000000 ) ) ;
#18055=LINE ( 'NONE', #3613, #716 ) ;
#18068=DIRECTION ( 'NONE',  ( -0.000000000000000000, 0.000000000000000000, 1.000000000000000000 ) ) ;
#18079=VECTOR ( 'NONE', #17789, 1000.000000000000000 ) ;
#18087=ORIENTED_EDGE ( 'NONE', *, *, #1570, .T. ) ;
#18107=DIRECTION ( 'NONE',  ( 0.000000000000000000, 0.8660254037844364872, 0.5000000000000036637 ) ) ;
#18112=DIRECTION ( 'NONE',  ( 0.000000000000000000, -0.8660254037844364872, -0.5000000000000036637 ) ) ;
#18136=ORIENTED_EDGE ( 'NONE', *, *, #858, .F. ) ;
#18150=ORIENTED_EDGE ( 'NONE', *, *, #5440, .T. ) ;
#18153=VECTOR ( 'NONE', #4904, 1000.000000000000000 ) ;
#18159=EDGE_LOOP ( 'NONE', ( #16526, #8538, #11228, #17935 ) ) ;
#18166=EDGE_CURVE ( 'NONE', #3797, #17800, #10322, .T. ) ;
#18167=LINE ( 'NONE', #13447, #5645 ) ;
#18204=CARTESIAN_POINT ( 'NONE',  ( 13.49999999999998401, -25.49999999999999645, 4.000000000000000000 ) ) ;
#18207=LINE ( 'NONE', #10247, #14322 ) ;
#18235=VERTEX_POINT ( 'NONE', #1009 ) ;
#18275=FACE_OUTER_BOUND ( 'NONE', #15954, .T. ) ;
#18314=EDGE_CURVE ( 'NONE', #483, #20175, #4288, .T. ) ;
#18356=VECTOR ( 'NONE', #15404, 1000.000000000000227 ) ;
#18374=ORIENTED_EDGE ( 'NONE', *, *, #1806, .F. ) ;
#18379=CARTESIAN_POINT ( 'NONE',  ( 11.00000000000000000, -20.16506350946107418, 5.000000000000000000 ) ) ;
#18381=CARTESIAN_POINT ( 'NONE',  ( 0.000000000000000000, 0.000000000000000000, 4.000000000000000000 ) ) ;
#18393=ORIENTED_EDGE ( 'NONE', *, *, #14183, .F. ) ;
#18394=LINE ( 'NONE', #15030, #7621 ) ;
#18396=VERTEX_POINT ( 'NONE', #18900 ) ;
#18401=EDGE_CURVE ( 'NONE', #17464, #16697, #9370, .T. ) ;
#18417=CARTESIAN_POINT ( 'NONE',  ( -2.499999999999998668, -19.50000000000000000, 1.000000000000000000 ) ) ;
#18447=ORIENTED_EDGE ( 'NONE', *, *, #10640, .T. ) ;
#18456=LINE ( 'NONE', #7670, #8364 ) ;
#18461=VERTEX_POINT ( 'NONE', #4657 ) ;
#18463=AXIS2_PLACEMENT_3D ( 'NONE', #4451, #19273, #4926 ) ;
#18507=ADVANCED_FACE ( 'NONE', ( #14484 ), #19000, .F. ) ;
#18517=DIRECTION ( 'NONE',  ( -1.000000000000000000, -0.000000000000000000, -0.000000000000000000 ) ) ;
#18523=EDGE_LOOP ( 'NONE', ( #18393, #3162, #2457, #5400 ) ) ;
#18531=DIRECTION ( 'NONE',  ( -0.000000000000000000, -1.000000000000000000, 0.000000000000000000 ) ) ;
#18570=DIRECTION ( 'NONE',  ( 0.000000000000000000, 0.000000000000000000, 1.000000000000000000 ) ) ;
#18572=ORIENTED_EDGE ( 'NONE', *, *, #13755, .T. ) ;
#18580=LINE ( 'NONE', #5821, #2641 ) ;
#18601=VERTEX_POINT ( 'NONE', #4863 ) ;
#18603=CARTESIAN_POINT ( 'NONE',  ( -3.499999999999997780, -24.49999999999999289, 1.000000000000000000 ) ) ;
#18619=EDGE_CURVE ( 'NONE', #4544, #7379, #6335, .T. ) ;
#18620=FACE_OUTER_BOUND ( 'NONE', #6935, .T. ) ;
#18628=DIRECTION ( 'NONE',  ( 0.000000000000000000, 0.000000000000000000, 1.000000000000000000 ) ) ;
#18639=CARTESIAN_POINT ( 'NONE',  ( 11.00000000000000000, -18.49999999999999645, 6.500000000000000888 ) ) ;
#18643=VERTEX_POINT ( 'NONE', #17517 ) ;
#18664=DIRECTION ( 'NONE',  ( -1.000000000000000000, -0.000000000000000000, -0.000000000000000000 ) ) ;
#18671=ORIENTED_EDGE ( 'NONE', *, *, #1030, .F. ) ;
#18676=ORIENTED_EDGE ( 'NONE', *, *, #5914, .F. ) ;
#18702=EDGE_CURVE ( 'NONE', #5682, #17800, #15101, .T. ) ;
#18716=DIRECTION ( 'NONE',  ( 0.000000000000000000, 0.000000000000000000, 1.000000000000000000 ) ) ;
#18722=CARTESIAN_POINT ( 'NONE',  ( 11.00000000000000000, -25.49999999999999645, 6.500000000000000000 ) ) ;
#18738=CARTESIAN_POINT ( 'NONE',  ( 7.499999999999999112, -18.49999999999999645, 6.500000000000000888 ) ) ;
#18755=DIRECTION ( 'NONE',  ( -1.000000000000000000, 0.000000000000000000, 0.000000000000000000 ) ) ;
#18757=AXIS2_PLACEMENT_3D ( 'NONE', #5246, #5355, #19391 ) ;
#18766=CARTESIAN_POINT ( 'NONE',  ( 7.499999999999999112, -20.16506350946107418, 5.250000000000000000 ) ) ;
#18771=VECTOR ( 'NONE', #2054, 1000.000000000000000 ) ;
#18778=ORIENTED_EDGE ( 'NONE', *, *, #20608, .T. ) ;
#18826=EDGE_LOOP ( 'NONE', ( #15190, #2385, #8789, #5760 ) ) ;
#18867=CARTESIAN_POINT ( 'NONE',  ( 3.499999999999998668, -19.50000000000000000, 1.000000000000000000 ) ) ;
#18871=EDGE_CURVE ( 'NONE', #20090, #9554, #2627, .T. ) ;
#18879=ORIENTED_EDGE ( 'NONE', *, *, #3482, .T. ) ;
#18891=EDGE_CURVE ( 'NONE', #15348, #9078, #1192, .T. ) ;
#18900=CARTESIAN_POINT ( 'NONE',  ( -14.49999999999998579, -21.99999999999999645, 12.00000000000000355 ) ) ;
#18908=ORIENTED_EDGE ( 'NONE', *, *, #10183, .F. ) ;
#18910=LINE ( 'NONE', #9274, #8981 ) ;
#18915=EDGE_LOOP ( 'NONE', ( #11992, #17175, #16225, #19764, #5133, #8557 ) ) ;
#18927=ORIENTED_EDGE ( 'NONE', *, *, #14910, .F. ) ;
#18931=ORIENTED_EDGE ( 'NONE', *, *, #17075, .F. ) ;
#18933=DIRECTION ( 'NONE',  ( -0.000000000000000000, 0.000000000000000000, -1.000000000000000000 ) ) ;
#18934=ORIENTED_EDGE ( 'NONE', *, *, #1360, .T. ) ;
#18935=CARTESIAN_POINT ( 'NONE',  ( 13.49999999999998401, -25.49999999999999645, 4.000000000000000000 ) ) ;
#18968=DIRECTION ( 'NONE',  ( 1.000000000000000000, -0.000000000000000000, -0.000000000000000000 ) ) ;
#18970=VECTOR ( 'NONE', #15790, 1000.000000000000000 ) ;
#18986=ORIENTED_EDGE ( 'NONE', *, *, #11038, .F. ) ;
#18991=ORIENTED_EDGE ( 'NONE', *, *, #2595, .F. ) ;
#18997=CARTESIAN_POINT ( 'NONE',  ( 14.49999999999998579, -21.99999999999999645, 11.68378559369222280 ) ) ;
#19000=PLANE ( 'NONE',  #8306 ) ;
#19020=CIRCLE ( 'NONE', #3295, 0.2500000000000002220 ) ;
#19039=CARTESIAN_POINT ( 'NONE',  ( 3.499999999999998668, -19.50000000000000000, 1.000000000000000000 ) ) ;
#19041=EDGE_LOOP ( 'NONE', ( #9558, #2561, #11233, #1534 ) ) ;
#19042=VECTOR ( 'NONE', #1327, 1000.000000000000000 ) ;
#19061=ORIENTED_EDGE ( 'NONE', *, *, #9798, .T. ) ;
#19099=CARTESIAN_POINT ( 'NONE',  ( 2.499999999999998668, -19.50000000000000000, 1.000000000000000000 ) ) ;
#19118=ORIENTED_EDGE ( 'NONE', *, *, #415, .F. ) ;
#19136=( NAMED_UNIT ( * ) SI_UNIT ( $, .STERADIAN. ) SOLID_ANGLE_UNIT ( ) );
#19141=ORIENTED_EDGE ( 'NONE', *, *, #18871, .T. ) ;
#19148=DIRECTION ( 'NONE',  ( 0.000000000000000000, 0.1264857625231113059, 0.9919684228235025047 ) ) ;
#19153=EDGE_CURVE ( 'NONE', #7462, #6837, #13498, .T. ) ;
#19164=VECTOR ( 'NONE', #2176, 1000.000000000000000 ) ;
#19165=EDGE_CURVE ( 'NONE', #8626, #8041, #9663, .T. ) ;
#19177=PRODUCT_DEFINITION ( 'UNKNOWN', '', #5035, #12560 ) ;
#19212=PRODUCT ( 'spring housing', 'spring housing', '', ( #6886 ) ) ;
#19218=VERTEX_POINT ( 'NONE', #18417 ) ;
#19221=ORIENTED_EDGE ( 'NONE', *, *, #1732, .F. ) ;
#19228=AXIS2_PLACEMENT_3D ( 'NONE', #13013, #3195, #10939 ) ;
#19229=EDGE_LOOP ( 'NONE', ( #9605, #9489, #17103, #1824 ) ) ;
#19234=CARTESIAN_POINT ( 'NONE',  ( -2.499999999999998668, -19.50000000000000000, 4.000000000000000000 ) ) ;
#19248=ORIENTED_EDGE ( 'NONE', *, *, #5501, .F. ) ;
#19256=FACE_OUTER_BOUND ( 'NONE', #18826, .T. ) ;
#19263=ADVANCED_FACE ( 'NONE', ( #8995 ), #5758, .F. ) ;
#19264=EDGE_CURVE ( 'NONE', #13151, #15413, #6904, .T. ) ;
#19273=DIRECTION ( 'NONE',  ( 1.000000000000000000, 0.000000000000000000, -0.000000000000000000 ) ) ;
#19280=ADVANCED_FACE ( 'NONE', ( #5337 ), #13272, .F. ) ;
#19291=AXIS2_PLACEMENT_3D ( 'NONE', #13416, #14882, #560 ) ;
#19357=EDGE_CURVE ( 'NONE', #17356, #13797, #18207, .T. ) ;
#19369=VECTOR ( 'NONE', #20586, 1000.000000000000000 ) ;
#19370=EDGE_CURVE ( 'NONE', #12022, #19576, #938, .T. ) ;
#19380=LINE ( 'NONE', #9636, #11690 ) ;
#19382=EDGE_CURVE ( 'NONE', #12385, #13259, #3970, .T. ) ;
#19388=DIRECTION ( 'NONE',  ( -1.000000000000000000, 0.000000000000000000, 0.000000000000000000 ) ) ;
#19391=DIRECTION ( 'NONE',  ( 1.000000000000000000, 0.000000000000000000, -0.000000000000000000 ) ) ;
#19415=LINE ( 'NONE', #4860, #12764 ) ;
#19416=VECTOR ( 'NONE', #993, 1000.000000000000000 ) ;
#19421=AXIS2_PLACEMENT_3D ( 'NONE', #1395, #17593, #12568 ) ;
#19432=ORIENTED_EDGE ( 'NONE', *, *, #16053, .T. ) ;
#19448=ORIENTED_EDGE ( 'NONE', *, *, #11038, .T. ) ;
#19468=DIRECTION ( 'NONE',  ( 0.000000000000000000, 0.000000000000000000, 1.000000000000000000 ) ) ;
#19486=FACE_OUTER_BOUND ( 'NONE', #8688, .T. ) ;
#19504=AXIS2_PLACEMENT_3D ( 'NONE', #2087, #8782, #5324 ) ;
#19513=DIRECTION ( 'NONE',  ( 0.000000000000000000, 0.000000000000000000, 1.000000000000000000 ) ) ;
#19529=ADVANCED_FACE ( 'NONE', ( #18620 ), #7629, .T. ) ;
#19541=CARTESIAN_POINT ( 'NONE',  ( -11.00000000000000000, -25.49999999999999645, 4.000000000000000000 ) ) ;
#19544=AXIS2_PLACEMENT_3D ( 'NONE', #16410, #16714, #14936 ) ;
#19564=FACE_OUTER_BOUND ( 'NONE', #17139, .T. ) ;
#19567=FACE_OUTER_BOUND ( 'NONE', #19229, .T. ) ;
#19576=VERTEX_POINT ( 'NONE', #4589 ) ;
#19589=DIRECTION ( 'NONE',  ( 0.000000000000000000, -1.000000000000000000, 0.000000000000000000 ) ) ;
#19592=DIRECTION ( 'NONE',  ( 0.000000000000000000, 0.000000000000000000, -1.000000000000000000 ) ) ;
#19610=CARTESIAN_POINT ( 'NONE',  ( 14.49999999999998579, -24.47992105705875332, 12.00000000000000000 ) ) ;
#19631=ORIENTED_EDGE ( 'NONE', *, *, #12096, .T. ) ;
#19668=DIRECTION ( 'NONE',  ( -1.000000000000000000, -0.000000000000000000, -0.000000000000000000 ) ) ;
#19677=LINE ( 'NONE', #8383, #7148 ) ;
#19710=AXIS2_PLACEMENT_3D ( 'NONE', #16414, #2089, #19468 ) ;
#19717=DIRECTION ( 'NONE',  ( -1.000000000000000000, -0.000000000000000000, -0.000000000000000000 ) ) ;
#19719=COLOUR_RGB ( '', 0.40784314, 0.44705882, 0.49803922) ;
#19734=ADVANCED_FACE ( 'NONE', ( #17556 ), #6788, .F. ) ;
#19735=ORIENTED_EDGE ( 'NONE', *, *, #10162, .F. ) ;
#19739=EDGE_CURVE ( 'NONE', #6837, #10229, #15879, .T. ) ;
#19757=ORIENTED_EDGE ( 'NONE', *, *, #1373, .T. ) ;
#19764=ORIENTED_EDGE ( 'NONE', *, *, #13431, .F. ) ;
#19773=FACE_BOUND ( 'NONE', #4395, .T. ) ;
#19774=VECTOR ( 'NONE', #623, 1000.000000000000000 ) ;
#19781=ORIENTED_EDGE ( 'NONE', *, *, #2352, .F. ) ;
#19782=DIRECTION ( 'NONE',  ( 0.000000000000000000, 0.000000000000000000, 1.000000000000000000 ) ) ;
#19783=FACE_OUTER_BOUND ( 'NONE', #19041, .T. ) ;
#19785=EDGE_CURVE ( 'NONE', #7462, #2297, #8252, .T. ) ;
#19787=ORIENTED_EDGE ( 'NONE', *, *, #570, .T. ) ;
#19838=ORIENTED_EDGE ( 'NONE', *, *, #11605, .F. ) ;
#19865=ORIENTED_EDGE ( 'NONE', *, *, #1709, .F. ) ;
#19877=EDGE_CURVE ( 'NONE', #18643, #12338, #12108, .T. ) ;
#19941=ORIENTED_EDGE ( 'NONE', *, *, #13480, .F. ) ;
#19970=DIRECTION ( 'NONE',  ( 0.000000000000000000, 1.000000000000000000, 0.000000000000000000 ) ) ;
#19982=CYLINDRICAL_SURFACE ( 'NONE', #12085, 1.000000000000002665 ) ;
#19995=VECTOR ( 'NONE', #8020, 1000.000000000000000 ) ;
#20022=AXIS2_PLACEMENT_3D ( 'NONE', #10109, #16485, #6564 ) ;
#20059=VECTOR ( 'NONE', #16214, 1000.000000000000000 ) ;
#20067=VERTEX_POINT ( 'NONE', #11231 ) ;
#20076=ORIENTED_EDGE ( 'NONE', *, *, #19370, .F. ) ;
#20080=CARTESIAN_POINT ( 'NONE',  ( -11.00000000000000000, -24.49999999999999289, 5.000000000000000000 ) ) ;
#20081=LINE ( 'NONE', #17336, #362 ) ;
#20082=LINE ( 'NONE', #7314, #7014 ) ;
#20088=EDGE_CURVE ( 'NONE', #17295, #5898, #13774, .T. ) ;
#20090=VERTEX_POINT ( 'NONE', #1508 ) ;
#20125=UNCERTAINTY_MEASURE_WITH_UNIT (LENGTH_MEASURE( 1.000000000000000082E-05 ), #6364, 'distance_accuracy_value', 'NONE');
#20140=EDGE_LOOP ( 'NONE', ( #19838, #19448, #17599, #18991 ) ) ;
#20142=CARTESIAN_POINT ( 'NONE',  ( 13.50000000000001243, -24.49999999999999289, 4.000000000000000000 ) ) ;
#20148=VERTEX_POINT ( 'NONE', #2694 ) ;
#20175=VERTEX_POINT ( 'NONE', #6632 ) ;
#20181=ORIENTED_EDGE ( 'NONE', *, *, #9898, .F. ) ;
#20195=CARTESIAN_POINT ( 'NONE',  ( -11.00000000000000000, -18.49999999999999645, 4.000000000000000000 ) ) ;
#20196=FACE_OUTER_BOUND ( 'NONE', #248, .T. ) ;
#20206=CARTESIAN_POINT ( 'NONE',  ( -11.00000000000000000, -23.83493649053891517, 5.249999999999999112 ) ) ;
#20210=DIRECTION ( 'NONE',  ( -1.000000000000000000, -0.000000000000000000, -0.000000000000000000 ) ) ;
#20223=VERTEX_POINT ( 'NONE', #354 ) ;
#20231=EDGE_CURVE ( 'NONE', #11513, #2226, #5257, .T. ) ;
#20232=DIRECTION ( 'NONE',  ( -0.000000000000000000, 1.000000000000000000, -0.000000000000000000 ) ) ;
#20250=FACE_OUTER_BOUND ( 'NONE', #10448, .T. ) ;
#20285=DIRECTION ( 'NONE',  ( -0.000000000000000000, 1.304178812473495102E-15, 1.000000000000000000 ) ) ;
#20294=CARTESIAN_POINT ( 'NONE',  ( -7.499999999999999112, -18.49999999999999645, 6.500000000000000888 ) ) ;
#20332=DIRECTION ( 'NONE',  ( 0.000000000000000000, 0.000000000000000000, 1.000000000000000000 ) ) ;
#20361=DIRECTION ( 'NONE',  ( -1.000000000000000000, -0.000000000000000000, -0.000000000000000000 ) ) ;
#20362=AXIS2_PLACEMENT_3D ( 'NONE', #1826, #17616, #8112 ) ;
#20390=LINE ( 'NONE', #15456, #13306 ) ;
#20393=PLANE ( 'NONE',  #8990 ) ;
#20394=DIRECTION ( 'NONE',  ( -8.673617379884047798E-17, 1.000000000000000000, -0.000000000000000000 ) ) ;
#20420=FACE_OUTER_BOUND ( 'NONE', #14099, .T. ) ;
#20425=CARTESIAN_POINT ( 'NONE',  ( 2.499999999999998668, -19.50000000000000000, 4.000000000000000000 ) ) ;
#20429=EDGE_CURVE ( 'NONE', #6686, #6562, #10387, .T. ) ;
#20440=CIRCLE ( 'NONE', #11396, 2.500000000000000444 ) ;
#20448=CARTESIAN_POINT ( 'NONE',  ( -11.00000000000000000, -20.16506350946107418, 5.000000000000000000 ) ) ;
#20449=DIRECTION ( 'NONE',  ( 1.000000000000000000, -0.000000000000000000, -0.000000000000000000 ) ) ;
#20468=EDGE_CURVE ( 'NONE', #12772, #20175, #8822, .T. ) ;
#20502=CARTESIAN_POINT ( 'NONE',  ( -11.00000000000000000, -24.49999999999999289, 4.000000000000000000 ) ) ;
#20506=PLANE ( 'NONE',  #17213 ) ;
#20510=LINE ( 'NONE', #8043, #2742 ) ;
#20517=( NAMED_UNIT ( * ) SI_UNIT ( $, .STERADIAN. ) SOLID_ANGLE_UNIT ( ) );
#20518=EDGE_LOOP ( 'NONE', ( #16398, #790, #2949, #13637 ) ) ;
#20521=DIRECTION ( 'NONE',  ( -1.000000000000000000, -0.000000000000000000, -0.000000000000000000 ) ) ;
#20548=CARTESIAN_POINT ( 'NONE',  ( -14.49999999999998579, -18.49999999999999645, 1.000000000000000000 ) ) ;
#20549=DIRECTION ( 'NONE',  ( -1.000000000000000000, -0.000000000000000000, -0.000000000000000000 ) ) ;
#20584=VERTEX_POINT ( 'NONE', #17267 ) ;
#20586=DIRECTION ( 'NONE',  ( 0.000000000000000000, 0.000000000000000000, 1.000000000000000000 ) ) ;
#20591=ADVANCED_FACE ( 'NONE', ( #2946 ), #1582, .T. ) ;
#20596=FACE_OUTER_BOUND ( 'NONE', #7713, .T. ) ;
#20608=EDGE_CURVE ( 'NONE', #2127, #5816, #3332, .T. ) ;
#20614=DIRECTION ( 'NONE',  ( 1.000000000000000000, -0.000000000000000000, 0.000000000000000000 ) ) ;
#20619=LINE ( 'NONE', #11394, #18970 ) ;
#20651=AXIS2_PLACEMENT_3D ( 'NONE', #735, #2715, #3964 ) ;
#20661=VERTEX_POINT ( 'NONE', #14648 ) ;
#20668=CARTESIAN_POINT ( 'NONE',  ( 7.499999999999999112, -19.49999999999999645, 5.000000000000000000 ) ) ;
#20671=DIRECTION ( 'NONE',  ( -0.000000000000000000, 1.000000000000000000, -1.304178812473495102E-15 ) ) ;
#20691=VECTOR ( 'NONE', #12423, 1000.000000000000000 ) ;
#20710=VECTOR ( 'NONE', #12805, 1000.000000000000000 ) ;
#20713=VECTOR ( 'NONE', #3800, 1000.000000000000000 ) ;
ENDSEC;
END-ISO-10303-21;
